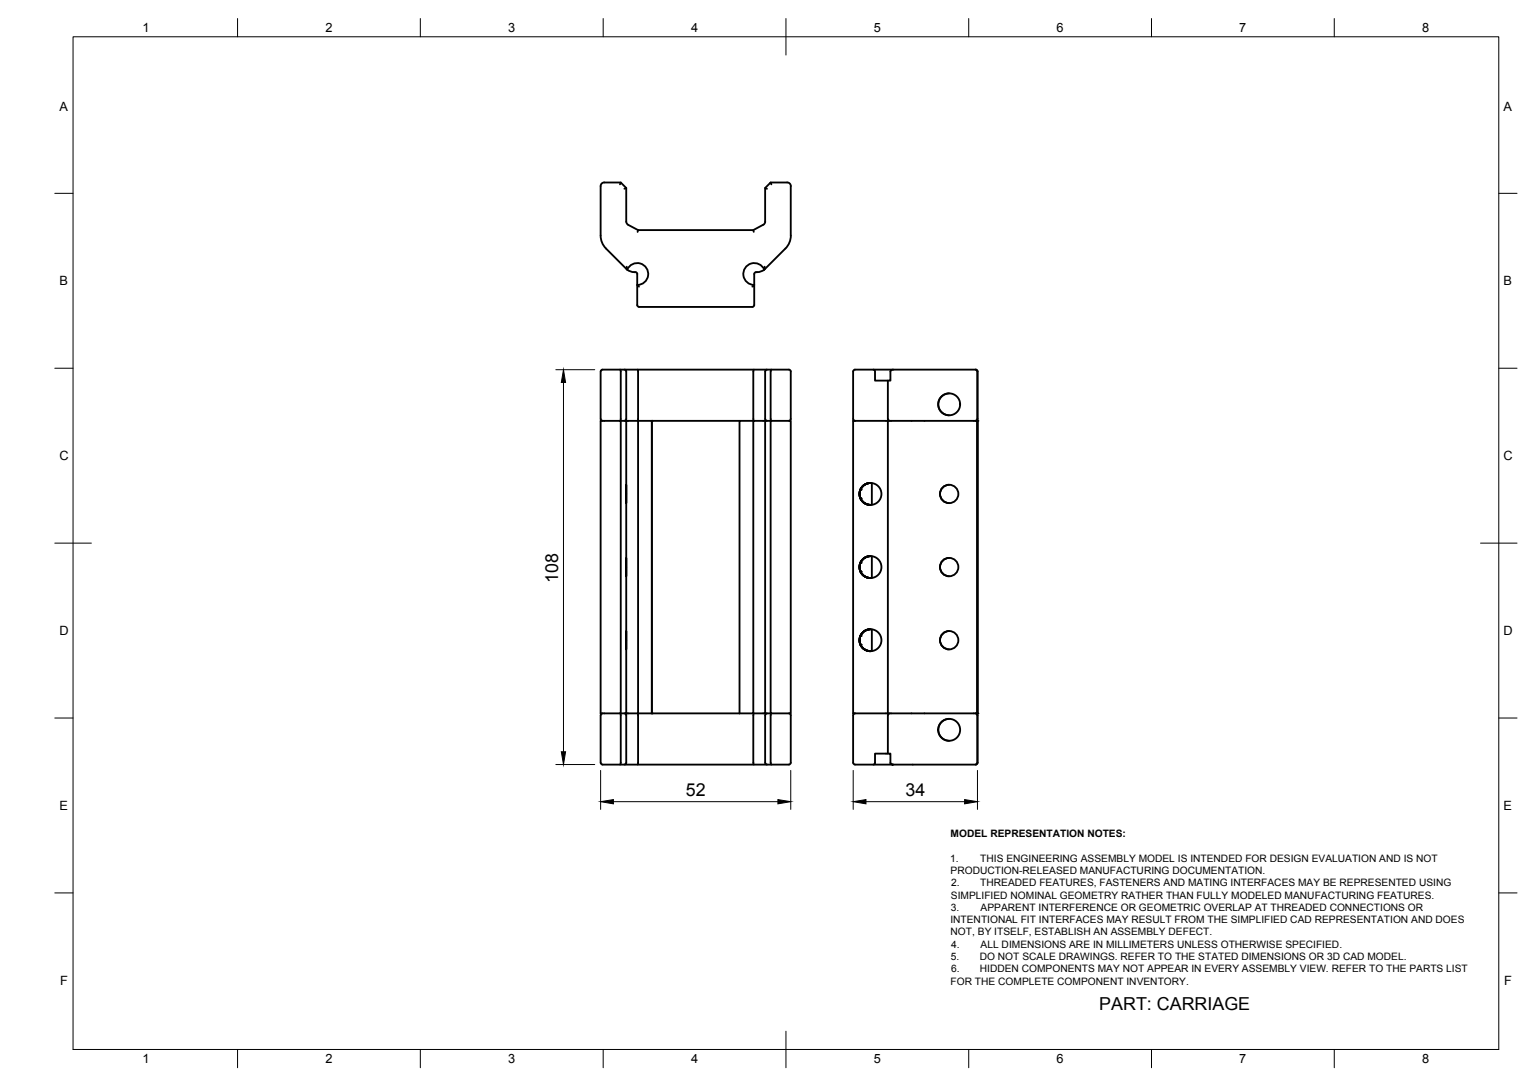
ISO-10303-21;
HEADER;
/* Generated by software containing ST-Developer
 * from STEP Tools, Inc. (www.steptools.com) 
 */

FILE_DESCRIPTION(
/* description */ (''),
/* implementation_level */ '2;1');

FILE_NAME(
/* name */ 'Carriage.step',
/* time_stamp */ '2026-10-05T11:01:41-07:00',
/* author */ (''),
/* organization */ (''),
/* preprocessor_version */ 'ST-DEVELOPER v20.2',
/* originating_system */ 'Autodesk Translation Framework v15.15.0.0',
/* authorisation */ '');

FILE_SCHEMA (('AUTOMOTIVE_DESIGN { 1 0 10303 214 3 1 1 }'));
ENDSEC;

DATA;
#10=MECHANICAL_DESIGN_GEOMETRIC_PRESENTATION_REPRESENTATION('',(#2142),#215609);
#119=ELLIPSE('',#29169,4.24264068711927,3.);
#120=ELLIPSE('',#29170,4.24264068711929,3.);
#121=ELLIPSE('',#29171,4.24264068711929,3.);
#122=ELLIPSE('',#29172,4.24279214221557,3.);
#123=ELLIPSE('',#29173,4.24279214221557,3.);
#124=ELLIPSE('',#29174,4.24248924824133,3.);
#125=ELLIPSE('',#29179,4.24248924824133,3.);
#126=ELLIPSE('',#29180,4.24279214221557,3.);
#127=ELLIPSE('',#29181,4.24264068711929,3.);
#128=ELLIPSE('',#29182,4.24264068711927,3.);
#129=ELLIPSE('',#29189,4.24264068711927,3.);
#130=ELLIPSE('',#29190,4.24264068711929,3.);
#131=ELLIPSE('',#29191,4.24264068711929,3.);
#132=ELLIPSE('',#29192,4.24279214221557,3.);
#133=ELLIPSE('',#29193,4.24279214221557,3.);
#134=ELLIPSE('',#29194,4.24248924824133,3.);
#135=ELLIPSE('',#29199,4.24248924824133,3.);
#136=ELLIPSE('',#29200,4.24279214221557,3.);
#137=ELLIPSE('',#29201,4.24264068711929,3.);
#138=ELLIPSE('',#29202,4.24264068711927,3.);
#139=ELLIPSE('',#29209,4.24264068711928,3.00000000000001);
#140=ELLIPSE('',#29210,4.24264068711931,3.00000000000001);
#141=ELLIPSE('',#29211,4.24264068711931,3.00000000000001);
#142=ELLIPSE('',#29212,4.24279214221559,3.00000000000001);
#143=ELLIPSE('',#29213,4.24279214221559,3.00000000000001);
#144=ELLIPSE('',#29214,4.24248924824134,3.00000000000001);
#145=ELLIPSE('',#29219,4.24248924824134,3.00000000000001);
#146=ELLIPSE('',#29220,4.24279214221559,3.00000000000001);
#147=ELLIPSE('',#29221,4.24264068711931,3.00000000000001);
#148=ELLIPSE('',#29222,4.24264068711928,3.00000000000001);
#204=FACE_BOUND('',#5046,.T.);
#205=FACE_BOUND('',#5047,.T.);
#206=FACE_BOUND('',#5048,.T.);
#207=FACE_BOUND('',#5055,.T.);
#208=FACE_BOUND('',#5056,.T.);
#209=FACE_BOUND('',#5057,.T.);
#210=FACE_BOUND('',#5062,.T.);
#211=FACE_BOUND('',#5063,.T.);
#212=FACE_BOUND('',#5064,.T.);
#213=FACE_BOUND('',#5089,.T.);
#214=FACE_BOUND('',#5090,.T.);
#215=FACE_BOUND('',#5091,.T.);
#1155=B_SPLINE_CURVE_WITH_KNOTS('',3,(#125658,#125659,#125660,#125661),
 .UNSPECIFIED.,.F.,.F.,(4,4),(0.425543658173478,0.45601992980538),
 .UNSPECIFIED.);
#1156=B_SPLINE_CURVE_WITH_KNOTS('',3,(#125665,#125666,#125667,#125668,#125669,
#125670,#125671,#125672,#125673,#125674),.UNSPECIFIED.,.F.,.F.,(4,2,2,2,
4),(-0.396099187348511,-0.387517388693499,-0.378935590038487,-0.34840050848607,
-0.288839883428953),.UNSPECIFIED.);
#1157=B_SPLINE_CURVE_WITH_KNOTS('',3,(#125678,#125679,#125680,#125681,#125682,
#125683,#125684,#125685,#125686,#125687,#125688,#125689,#125690,#125691,
#125692,#125693,#125694,#125695,#125696,#125697,#125698,#125699,#125700,
#125701,#125702,#125703),.UNSPECIFIED.,.F.,.F.,(4,2,2,2,2,2,2,2,2,2,2,2,
4),(0.255174199615659,0.258977839880058,0.262781480144458,0.270388760673256,
0.281246247196537,0.307084793231223,0.382761299423499,0.458437805615774,
0.484276351650461,0.495133838173742,0.50274111870254,0.506544758966939,
0.510348399231339),.UNSPECIFIED.);
#1158=B_SPLINE_CURVE_WITH_KNOTS('',3,(#125707,#125708,#125709,#125710,#125711,
#125712,#125713,#125714,#125715,#125716),.UNSPECIFIED.,.F.,.F.,(4,2,2,2,
4),(-0.107259303919562,-0.047698678862445,-0.0171635973100282,-0.00858179865501664,
-5.10702591327572E-15),.UNSPECIFIED.);
#1159=B_SPLINE_CURVE_WITH_KNOTS('',3,(#125720,#125721,#125722,#125723,#125724,
#125725),.UNSPECIFIED.,.F.,.F.,(4,2,4),(-0.229255666072561,-0.191461818559235,
-0.153667971045909),.UNSPECIFIED.);
#1160=B_SPLINE_CURVE_WITH_KNOTS('',3,(#125729,#125730,#125731,#125732,#125733,
#125734),.UNSPECIFIED.,.F.,.F.,(4,2,4),(-0.629374586597435,-0.551502061005561,
-0.473629535413688),.UNSPECIFIED.);
#1161=B_SPLINE_CURVE_WITH_KNOTS('',3,(#125738,#125739,#125740,#125741,#125742,
#125743),.UNSPECIFIED.,.F.,.F.,(4,2,4),(-2.19173462068589,-2.01009835047604,
-1.80563850045614),.UNSPECIFIED.);
#1162=B_SPLINE_CURVE_WITH_KNOTS('',3,(#125747,#125748,#125749,#125750,#125751,
#125752,#125753,#125754,#125755,#125756,#125757,#125758,#125759,#125760,
#125761,#125762),.UNSPECIFIED.,.F.,.F.,(4,2,2,2,2,2,2,4),(-0.591143586973193,
-0.574347005517868,-0.557550424062543,-0.523957261151894,-0.475997826184756,
-0.428038391217618,-0.391437431812971,-0.357248738805367),.UNSPECIFIED.);
#1163=B_SPLINE_CURVE_WITH_KNOTS('',3,(#125766,#125767,#125768,#125769,#125770,
#125771,#125772,#125773,#125774,#125775,#125776,#125777,#125778,#125779,
#125780,#125781,#125782,#125783,#125784,#125785,#125786,#125787,#125788,
#125789,#125790,#125791),.UNSPECIFIED.,.F.,.F.,(4,2,2,2,2,2,2,2,2,2,2,2,
4),(0.,0.00380879604231436,0.00761759208462871,0.0152351841692574,0.0261059417541897,
0.0519747072078825,0.127764798734132,0.203554890260381,0.229423655714074,
0.240294413299006,0.247912005383635,0.251720801425949,0.255529597468264),
 .UNSPECIFIED.);
#1164=B_SPLINE_CURVE_WITH_KNOTS('',3,(#125795,#125796,#125797,#125798,#125799,
#125800,#125801,#125802,#125803,#125804,#125805,#125806,#125807,#125808,
#125809,#125810),.UNSPECIFIED.,.F.,.F.,(4,2,2,2,2,2,2,4),(-0.233894848167829,
-0.199706155160222,-0.163105195755574,-0.115145760788437,-0.0671863258212992,
-0.0335931629106496,-0.0167965814553248,0.),.UNSPECIFIED.);
#1165=B_SPLINE_CURVE_WITH_KNOTS('',3,(#125818,#125819,#125820,#125821,#125822,
#125823,#125824,#125825,#125826,#125827,#125828,#125829,#125830,#125831,
#125832,#125833),.UNSPECIFIED.,.F.,.F.,(4,2,2,2,2,2,2,4),(-0.295589574301039,
-0.278794522803568,-0.261996615556423,-0.228400801062134,-0.180435395401912,
-0.13246998974169,-0.0958671986171408,-0.0616743717891369),
 .UNSPECIFIED.);
#1166=B_SPLINE_CURVE_WITH_KNOTS('',3,(#125837,#125838,#125839,#125840,#125841,
#125842,#125843,#125844,#125845,#125846,#125847,#125848,#125849,#125850,
#125851,#125852,#125853,#125854,#125855,#125856,#125857,#125858,#125859,
#125860,#125861,#125862),.UNSPECIFIED.,.F.,.F.,(4,2,2,2,2,2,2,2,2,2,2,2,
4),(0.255403168241683,0.259209043849209,0.263015990348529,0.270629883347168,
0.281495880894667,0.307353808398232,0.383103146024835,0.458852483651438,
0.484710411155003,0.495576408702502,0.503190301701141,0.506997248200461,
0.510803123807987),.UNSPECIFIED.);
#1167=B_SPLINE_CURVE_WITH_KNOTS('',3,(#125866,#125867,#125868,#125869,#125870,
#125871,#125872,#125873,#125874,#125875,#125876,#125877,#125878,#125879,
#125880,#125881),.UNSPECIFIED.,.F.,.F.,(4,2,2,2,2,2,2,4),(-0.525961887431026,
-0.491769060603023,-0.455166269478473,-0.407200863818251,-0.35923545815803,
-0.32563964366374,-0.308841736416595,-0.292046684919125),.UNSPECIFIED.);
#1168=B_SPLINE_CURVE_WITH_KNOTS('',3,(#125885,#125886,#125887,#125888,#125889,
#125890,#125891,#125892),.UNSPECIFIED.,.F.,.F.,(4,2,2,4),(-1.80557842881869,
-1.80556058066602,-1.60110476302328,-1.41948692443241),.UNSPECIFIED.);
#1169=B_SPLINE_CURVE_WITH_KNOTS('',3,(#125896,#125897,#125898,#125899,#125900,
#125901),.UNSPECIFIED.,.F.,.F.,(4,2,4),(-0.15576381568435,-0.0783128305768447,
-7.13925426615558E-6),.UNSPECIFIED.);
#1170=B_SPLINE_CURVE_WITH_KNOTS('',3,(#125905,#125906,#125907,#125908,#125909,
#125910,#125911,#125912,#125913,#125914),.UNSPECIFIED.,.F.,.F.,(4,2,2,2,
4),(-0.151179644005164,-0.151176055112586,-0.113501375709474,-0.0758266963063619,
-0.0755936744236418),.UNSPECIFIED.);
#1171=B_SPLINE_CURVE_WITH_KNOTS('',3,(#125918,#125919,#125920,#125921,#125922,
#125923,#125924,#125925,#125926,#125927,#125928,#125929,#125930,#125931),
 .UNSPECIFIED.,.F.,.F.,(4,2,2,2,2,2,4),(-0.199196015359092,-0.199194230558666,
-0.188883836185403,-0.17857344181214,-0.157952653065614,-0.123832754584569,
-0.0897155491016723),.UNSPECIFIED.);
#1172=B_SPLINE_CURVE_WITH_KNOTS('',3,(#125935,#125936,#125937,#125938,#125939,
#125940,#125941,#125942,#125943,#125944,#125945,#125946,#125947,#125948,
#125949,#125950,#125951,#125952,#125953,#125954,#125955,#125956,#125957,
#125958,#125959,#125960,#125961,#125962,#125963,#125964,#125965),
 .UNSPECIFIED.,.F.,.F.,(4,3,2,2,2,2,2,2,2,2,2,2,2,2,4),(0.509893253687354,
0.509894324579146,0.513694670705264,0.517495016831383,0.525095709083619,
0.535944713171104,0.561763938973776,0.637367905723932,0.712971872474088,
0.73879109827676,0.749640102364244,0.757240794616481,0.7610411407426,0.764841486868718,
0.764842557760511),.UNSPECIFIED.);
#1173=B_SPLINE_CURVE_WITH_KNOTS('',3,(#125969,#125970,#125971,#125972,#125973,
#125974,#125975,#125976,#125977,#125978,#125979,#125980,#125981,#125982),
 .UNSPECIFIED.,.F.,.F.,(4,2,2,2,2,2,4),(-0.306485394370277,-0.272368188887381,
-0.238248290406335,-0.217627501659809,-0.207317107286546,-0.197006712913283,
-0.197004928112857),.UNSPECIFIED.);
#1174=B_SPLINE_CURVE_WITH_KNOTS('',3,(#125986,#125987,#125988,#125989,#125990,
#125991),.UNSPECIFIED.,.F.,.F.,(4,2,4),(-0.489035198690406,-0.458517781350602,
-0.458514192458025),.UNSPECIFIED.);
#1175=B_SPLINE_CURVE_WITH_KNOTS('',3,(#125997,#125998,#125999,#126000,#126001,
#126002,#126003,#126004),.UNSPECIFIED.,.F.,.F.,(4,2,2,4),(-0.534100162039546,
-0.533867140156826,-0.496192460753714,-0.489035198690406),.UNSPECIFIED.);
#1176=B_SPLINE_CURVE_WITH_KNOTS('',3,(#126008,#126009,#126010,#126011,#126012,
#126013),.UNSPECIFIED.,.F.,.F.,(4,2,4),(-1.25873888352118,-1.1804331921986,
-1.10298220709109),.UNSPECIFIED.);
#1177=B_SPLINE_CURVE_WITH_KNOTS('',3,(#126017,#126018,#126019,#126020,#126021,
#126022,#126023,#126024,#126025),.UNSPECIFIED.,.F.,.F.,(4,2,3,4),(-0.386073656233604,
-0.204455817642737,0.,1.78481526716903E-5),.UNSPECIFIED.);
#1178=B_SPLINE_CURVE_WITH_KNOTS('',3,(#126030,#126031,#126032,#126033,#126034,
#126035),.UNSPECIFIED.,.F.,.F.,(4,2,4),(-3.61127700091229,-3.40681715089239,
-3.22518088068254),.UNSPECIFIED.);
#1179=B_SPLINE_CURVE_WITH_KNOTS('',3,(#126039,#126040,#126041,#126042,#126043,
#126044),.UNSPECIFIED.,.F.,.F.,(4,2,4),(-0.785102654344136,-0.707230128752262,
-0.629357603160389),.UNSPECIFIED.);
#1180=B_SPLINE_CURVE_WITH_KNOTS('',3,(#126047,#126048,#126049,#126050,#126051,
#126052),.UNSPECIFIED.,.F.,.F.,(4,2,4),(0.380432234778735,0.418226082292058,
0.425543658173478),.UNSPECIFIED.);
#1181=B_SPLINE_CURVE_WITH_KNOTS('',3,(#126064,#126065,#126066,#126067),
 .UNSPECIFIED.,.F.,.F.,(4,4),(0.425543658173478,0.45601992980538),
 .UNSPECIFIED.);
#1182=B_SPLINE_CURVE_WITH_KNOTS('',3,(#126071,#126072,#126073,#126074,#126075,
#126076,#126077,#126078,#126079,#126080),.UNSPECIFIED.,.F.,.F.,(4,2,2,2,
4),(-0.396099187348511,-0.387517388693499,-0.378935590038488,-0.348400508486071,
-0.288839883428954),.UNSPECIFIED.);
#1183=B_SPLINE_CURVE_WITH_KNOTS('',3,(#126084,#126085,#126086,#126087,#126088,
#126089,#126090,#126091,#126092,#126093,#126094,#126095,#126096,#126097,
#126098,#126099,#126100,#126101,#126102,#126103,#126104,#126105,#126106,
#126107,#126108,#126109),.UNSPECIFIED.,.F.,.F.,(4,2,2,2,2,2,2,2,2,2,2,2,
4),(0.255174199615659,0.258977839880058,0.262781480144457,0.270388760673256,
0.281246247196536,0.307084793231223,0.382761299423499,0.458437805615774,
0.48427635165046,0.495133838173741,0.50274111870254,0.506544758966939,0.510348399231338),
 .UNSPECIFIED.);
#1184=B_SPLINE_CURVE_WITH_KNOTS('',3,(#126113,#126114,#126115,#126116,#126117,
#126118,#126119,#126120,#126121,#126122),.UNSPECIFIED.,.F.,.F.,(4,2,2,2,
4),(-0.107259303919562,-0.047698678862445,-0.0171635973100282,-0.00858179865501664,
-5.10702591327572E-15),.UNSPECIFIED.);
#1185=B_SPLINE_CURVE_WITH_KNOTS('',3,(#126126,#126127,#126128,#126129,#126130,
#126131),.UNSPECIFIED.,.F.,.F.,(4,2,4),(-0.229255666072561,-0.191461818559235,
-0.153667971045909),.UNSPECIFIED.);
#1186=B_SPLINE_CURVE_WITH_KNOTS('',3,(#126135,#126136,#126137,#126138,#126139,
#126140),.UNSPECIFIED.,.F.,.F.,(4,2,4),(-0.629374586597435,-0.551502061005562,
-0.47362953541369),.UNSPECIFIED.);
#1187=B_SPLINE_CURVE_WITH_KNOTS('',3,(#126144,#126145,#126146,#126147,#126148,
#126149),.UNSPECIFIED.,.F.,.F.,(4,2,4),(-2.19173462068589,-2.01009835047603,
-1.80563850045614),.UNSPECIFIED.);
#1188=B_SPLINE_CURVE_WITH_KNOTS('',3,(#126153,#126154,#126155,#126156,#126157,
#126158,#126159,#126160,#126161,#126162,#126163,#126164,#126165,#126166,
#126167,#126168),.UNSPECIFIED.,.F.,.F.,(4,2,2,2,2,2,2,4),(-0.591143586973193,
-0.574347005517868,-0.557550424062543,-0.523957261151894,-0.475997826184756,
-0.428038391217618,-0.391437431812971,-0.357248738805362),.UNSPECIFIED.);
#1189=B_SPLINE_CURVE_WITH_KNOTS('',3,(#126172,#126173,#126174,#126175,#126176,
#126177,#126178,#126179,#126180,#126181,#126182,#126183,#126184,#126185,
#126186,#126187,#126188,#126189,#126190,#126191,#126192,#126193,#126194,
#126195,#126196,#126197),.UNSPECIFIED.,.F.,.F.,(4,2,2,2,2,2,2,2,2,2,2,2,
4),(0.,0.00380879604231436,0.00761759208462871,0.0152351841692574,0.0261059417541897,
0.0519747072078817,0.127764798734132,0.203554890260381,0.229423655714074,
0.240294413299006,0.247912005383635,0.251720801425949,0.255529597468264),
 .UNSPECIFIED.);
#1190=B_SPLINE_CURVE_WITH_KNOTS('',3,(#126201,#126202,#126203,#126204,#126205,
#126206,#126207,#126208,#126209,#126210,#126211,#126212,#126213,#126214,
#126215,#126216),.UNSPECIFIED.,.F.,.F.,(4,2,2,2,2,2,2,4),(-0.233894848167831,
-0.199706155160222,-0.163105195755574,-0.115145760788437,-0.0671863258212992,
-0.0335931629106496,-0.0167965814553248,0.),.UNSPECIFIED.);
#1191=B_SPLINE_CURVE_WITH_KNOTS('',3,(#126224,#126225,#126226,#126227,#126228,
#126229,#126230,#126231,#126232,#126233,#126234,#126235,#126236,#126237,
#126238,#126239),.UNSPECIFIED.,.F.,.F.,(4,2,2,2,2,2,2,4),(-0.295589574301039,
-0.278794522803568,-0.261996615556423,-0.228400801062134,-0.180435395401912,
-0.13246998974169,-0.0958671986171408,-0.0616743717891374),
 .UNSPECIFIED.);
#1192=B_SPLINE_CURVE_WITH_KNOTS('',3,(#126243,#126244,#126245,#126246,#126247,
#126248,#126249,#126250,#126251,#126252,#126253,#126254,#126255,#126256,
#126257,#126258,#126259,#126260,#126261,#126262,#126263,#126264,#126265,
#126266,#126267,#126268),.UNSPECIFIED.,.F.,.F.,(4,2,2,2,2,2,2,2,2,2,2,2,
4),(0.255403168241683,0.259209043849209,0.263015990348529,0.270629883347168,
0.281495880894667,0.307353808398233,0.383103146024836,0.458852483651437,
0.484710411155004,0.495576408702501,0.503190301701141,0.50699724820046,
0.510803123807986),.UNSPECIFIED.);
#1193=B_SPLINE_CURVE_WITH_KNOTS('',3,(#126272,#126273,#126274,#126275,#126276,
#126277,#126278,#126279,#126280,#126281,#126282,#126283,#126284,#126285,
#126286,#126287),.UNSPECIFIED.,.F.,.F.,(4,2,2,2,2,2,2,4),(-0.525961887431026,
-0.491769060603023,-0.455166269478473,-0.407200863818251,-0.35923545815803,
-0.32563964366374,-0.308841736416595,-0.292046684919125),.UNSPECIFIED.);
#1194=B_SPLINE_CURVE_WITH_KNOTS('',3,(#126291,#126292,#126293,#126294,#126295,
#126296,#126297,#126298),.UNSPECIFIED.,.F.,.F.,(4,2,2,4),(-1.80557842881869,
-1.80556058066602,-1.60110476302328,-1.41948692443241),.UNSPECIFIED.);
#1195=B_SPLINE_CURVE_WITH_KNOTS('',3,(#126302,#126303,#126304,#126305,#126306,
#126307),.UNSPECIFIED.,.F.,.F.,(4,2,4),(-0.15576381568435,-0.0783128305768447,
-7.13925426615561E-6),.UNSPECIFIED.);
#1196=B_SPLINE_CURVE_WITH_KNOTS('',3,(#126311,#126312,#126313,#126314,#126315,
#126316,#126317,#126318,#126319,#126320),.UNSPECIFIED.,.F.,.F.,(4,2,2,2,
4),(-0.151179644005162,-0.151176055112586,-0.113501375709474,-0.0758266963063619,
-0.0755936744236418),.UNSPECIFIED.);
#1197=B_SPLINE_CURVE_WITH_KNOTS('',3,(#126324,#126325,#126326,#126327,#126328,
#126329,#126330,#126331,#126332,#126333,#126334,#126335,#126336,#126337),
 .UNSPECIFIED.,.F.,.F.,(4,2,2,2,2,2,4),(-0.199196015359092,-0.199194230558666,
-0.188883836185403,-0.17857344181214,-0.157952653065614,-0.123832754584569,
-0.0897155491016734),.UNSPECIFIED.);
#1198=B_SPLINE_CURVE_WITH_KNOTS('',3,(#126341,#126342,#126343,#126344,#126345,
#126346,#126347,#126348,#126349,#126350,#126351,#126352,#126353,#126354,
#126355,#126356,#126357,#126358,#126359,#126360,#126361,#126362,#126363,
#126364,#126365,#126366,#126367,#126368,#126369,#126370,#126371),
 .UNSPECIFIED.,.F.,.F.,(4,3,2,2,2,2,2,2,2,2,2,2,2,2,4),(0.509893253687354,
0.509894324579146,0.513694670705264,0.517495016831383,0.525095709083619,
0.535944713171104,0.561763938973776,0.637367905723932,0.712971872474088,
0.73879109827676,0.749640102364244,0.757240794616481,0.7610411407426,0.764841486868718,
0.764842557760511),.UNSPECIFIED.);
#1199=B_SPLINE_CURVE_WITH_KNOTS('',3,(#126375,#126376,#126377,#126378,#126379,
#126380,#126381,#126382,#126383,#126384,#126385,#126386,#126387,#126388),
 .UNSPECIFIED.,.F.,.F.,(4,2,2,2,2,2,4),(-0.306485394370277,-0.272368188887381,
-0.238248290406335,-0.217627501659809,-0.207317107286546,-0.197006712913283,
-0.197004928112857),.UNSPECIFIED.);
#1200=B_SPLINE_CURVE_WITH_KNOTS('',3,(#126392,#126393,#126394,#126395,#126396,
#126397),.UNSPECIFIED.,.F.,.F.,(4,2,4),(-0.489035198690406,-0.458517781350602,
-0.458514192458025),.UNSPECIFIED.);
#1201=B_SPLINE_CURVE_WITH_KNOTS('',3,(#126403,#126404,#126405,#126406,#126407,
#126408,#126409,#126410),.UNSPECIFIED.,.F.,.F.,(4,2,2,4),(-0.534100162039546,
-0.533867140156826,-0.496192460753714,-0.489035198690406),.UNSPECIFIED.);
#1202=B_SPLINE_CURVE_WITH_KNOTS('',3,(#126414,#126415,#126416,#126417,#126418,
#126419),.UNSPECIFIED.,.F.,.F.,(4,2,4),(-1.25873888352118,-1.1804331921986,
-1.10298220709109),.UNSPECIFIED.);
#1203=B_SPLINE_CURVE_WITH_KNOTS('',3,(#126423,#126424,#126425,#126426,#126427,
#126428,#126429,#126430,#126431),.UNSPECIFIED.,.F.,.F.,(4,2,3,4),(-0.386073656233604,
-0.204455817642737,0.,1.78481526716903E-5),.UNSPECIFIED.);
#1204=B_SPLINE_CURVE_WITH_KNOTS('',3,(#126436,#126437,#126438,#126439,#126440,
#126441),.UNSPECIFIED.,.F.,.F.,(4,2,4),(-3.61127700091229,-3.40681715089239,
-3.22518088068254),.UNSPECIFIED.);
#1205=B_SPLINE_CURVE_WITH_KNOTS('',3,(#126445,#126446,#126447,#126448,#126449,
#126450),.UNSPECIFIED.,.F.,.F.,(4,2,4),(-0.785102654344136,-0.707230128752262,
-0.629357603160389),.UNSPECIFIED.);
#1206=B_SPLINE_CURVE_WITH_KNOTS('',3,(#126453,#126454,#126455,#126456,#126457,
#126458),.UNSPECIFIED.,.F.,.F.,(4,2,4),(0.380432234778735,0.418226082292058,
0.425543658173478),.UNSPECIFIED.);
#1207=B_SPLINE_CURVE_WITH_KNOTS('',3,(#126470,#126471,#126472,#126473),
 .UNSPECIFIED.,.F.,.F.,(4,4),(0.425543658173479,0.45601992980538),
 .UNSPECIFIED.);
#1208=B_SPLINE_CURVE_WITH_KNOTS('',3,(#126477,#126478,#126479,#126480,#126481,
#126482,#126483,#126484,#126485,#126486,#126487,#126488),.UNSPECIFIED.,
 .F.,.F.,(4,2,2,2,2,4),(-0.398283608397278,-0.387975515458133,-0.377667422518988,
-0.357051236640699,-0.322947181787487,-0.288843126934276),.UNSPECIFIED.);
#1209=B_SPLINE_CURVE_WITH_KNOTS('',3,(#126492,#126493,#126494,#126495,#126496,
#126497,#126498,#126499,#126500,#126501,#126502,#126503,#126504,#126505,
#126506,#126507,#126508,#126509,#126510,#126511,#126512,#126513,#126514,
#126515,#126516,#126517),.UNSPECIFIED.,.F.,.F.,(4,2,2,2,2,2,2,2,2,2,2,2,
4),(0.255174199615664,0.258977839880064,0.262781480144463,0.270388760673262,
0.281246247196542,0.307084793231227,0.382761299423505,0.458437805615783,
0.484276351650471,0.495133838173751,0.50274111870255,0.50654475896695,0.510348399231349),
 .UNSPECIFIED.);
#1210=B_SPLINE_CURVE_WITH_KNOTS('',3,(#126521,#126522,#126523,#126524,#126525,
#126526,#126527,#126528,#126529,#126530,#126531,#126532),.UNSPECIFIED.,
 .F.,.F.,(4,2,2,2,2,4),(-0.109440481463008,-0.075336426609796,-0.0412323717565842,
-0.0206161858782945,-0.0103080929391497,-4.88498130835069E-15),
 .UNSPECIFIED.);
#1211=B_SPLINE_CURVE_WITH_KNOTS('',3,(#126536,#126537,#126538,#126539,#126540,
#126541),.UNSPECIFIED.,.F.,.F.,(4,2,4),(-0.229255666072554,-0.191461818559231,
-0.153667971045908),.UNSPECIFIED.);
#1212=B_SPLINE_CURVE_WITH_KNOTS('',3,(#126545,#126546,#126547,#126548,#126549,
#126550),.UNSPECIFIED.,.F.,.F.,(4,2,4),(-0.629374586597435,-0.551502061005562,
-0.473629535413688),.UNSPECIFIED.);
#1213=B_SPLINE_CURVE_WITH_KNOTS('',3,(#126554,#126555,#126556,#126557,#126558,
#126559),.UNSPECIFIED.,.F.,.F.,(4,2,4),(-2.19173462068589,-2.01009835047604,
-1.80563850045615),.UNSPECIFIED.);
#1214=B_SPLINE_CURVE_WITH_KNOTS('',3,(#126563,#126564,#126565,#126566,#126567,
#126568,#126569,#126570,#126571,#126572,#126573,#126574,#126575,#126576,
#126577,#126578),.UNSPECIFIED.,.F.,.F.,(4,2,2,2,2,2,2,4),(-0.591143586973191,
-0.574347005517867,-0.557550424062542,-0.523957261151894,-0.475997826184755,
-0.428038391217617,-0.391437431812969,-0.357248738805361),.UNSPECIFIED.);
#1215=B_SPLINE_CURVE_WITH_KNOTS('',3,(#126582,#126583,#126584,#126585,#126586,
#126587,#126588,#126589,#126590,#126591,#126592,#126593,#126594,#126595,
#126596,#126597,#126598,#126599,#126600,#126601,#126602,#126603,#126604,
#126605,#126606,#126607),.UNSPECIFIED.,.F.,.F.,(4,2,2,2,2,2,2,2,2,2,2,2,
4),(0.,0.00380879604231454,0.00761759208462907,0.0152351841692581,0.0261059417541897,
0.0519747072078822,0.127764798734136,0.203554890260386,0.22942365571408,
0.240294413299011,0.24791200538364,0.251720801425955,0.255529597468269),
 .UNSPECIFIED.);
#1216=B_SPLINE_CURVE_WITH_KNOTS('',3,(#126611,#126612,#126613,#126614,#126615,
#126616,#126617,#126618,#126619,#126620,#126621,#126622,#126623,#126624,
#126625,#126626),.UNSPECIFIED.,.F.,.F.,(4,2,2,2,2,2,2,4),(-0.233894848167828,
-0.199706155160221,-0.163105195755574,-0.115145760788435,-0.0671863258212968,
-0.0335931629106484,-0.0167965814553242,0.),.UNSPECIFIED.);
#1217=B_SPLINE_CURVE_WITH_KNOTS('',3,(#126634,#126635,#126636,#126637,#126638,
#126639,#126640,#126641,#126642,#126643,#126644,#126645,#126646,#126647,
#126648,#126649),.UNSPECIFIED.,.F.,.F.,(4,2,2,2,2,2,2,4),(-0.295589574301038,
-0.278794522803567,-0.261996615556422,-0.228400801062133,-0.180435395401912,
-0.132469989741691,-0.095867198617141,-0.0616743717891376),
 .UNSPECIFIED.);
#1218=B_SPLINE_CURVE_WITH_KNOTS('',3,(#126653,#126654,#126655,#126656,#126657,
#126658,#126659,#126660,#126661,#126662,#126663,#126664,#126665,#126666,
#126667,#126668,#126669,#126670,#126671,#126672,#126673,#126674,#126675,
#126676,#126677,#126678),.UNSPECIFIED.,.F.,.F.,(4,2,2,2,2,2,2,2,2,2,2,2,
4),(0.255403168241688,0.259209043849214,0.263015990348534,0.270629883347173,
0.281495880894669,0.307353808398237,0.38310314602484,0.458852483651447,
0.484710411155011,0.495576408702511,0.50319030170115,0.506997248200469,
0.510803123807995),.UNSPECIFIED.);
#1219=B_SPLINE_CURVE_WITH_KNOTS('',3,(#126682,#126683,#126684,#126685,#126686,
#126687,#126688,#126689,#126690,#126691,#126692,#126693,#126694,#126695,
#126696,#126697),.UNSPECIFIED.,.F.,.F.,(4,2,2,2,2,2,2,4),(-0.525961887431025,
-0.491769060603021,-0.455166269478471,-0.40720086381825,-0.359235458158029,
-0.32563964366374,-0.308841736416595,-0.292046684919124),.UNSPECIFIED.);
#1220=B_SPLINE_CURVE_WITH_KNOTS('',3,(#126701,#126702,#126703,#126704,#126705,
#126706,#126707,#126708),.UNSPECIFIED.,.F.,.F.,(4,2,2,4),(-1.80557842881869,
-1.80556058066602,-1.60110476302328,-1.41948692443242),.UNSPECIFIED.);
#1221=B_SPLINE_CURVE_WITH_KNOTS('',3,(#126712,#126713,#126714,#126715,#126716,
#126717),.UNSPECIFIED.,.F.,.F.,(4,2,4),(-0.155763815684349,-0.0783128305768452,
-7.13925426615562E-6),.UNSPECIFIED.);
#1222=B_SPLINE_CURVE_WITH_KNOTS('',3,(#126721,#126722,#126723,#126724,#126725,
#126726,#126727,#126728,#126729,#126730),.UNSPECIFIED.,.F.,.F.,(4,2,2,2,
4),(-0.151179644004872,-0.151176055112587,-0.113501375709475,-0.0758266963063625,
-0.0755936744236423),.UNSPECIFIED.);
#1223=B_SPLINE_CURVE_WITH_KNOTS('',3,(#126734,#126735,#126736,#126737,#126738,
#126739,#126740,#126741,#126742,#126743,#126744,#126745,#126746,#126747),
 .UNSPECIFIED.,.F.,.F.,(4,2,2,2,2,2,4),(-0.199196015359092,-0.199194230558666,
-0.188883836185403,-0.178573441812139,-0.157952653065613,-0.123832754584568,
-0.0897155491016729),.UNSPECIFIED.);
#1224=B_SPLINE_CURVE_WITH_KNOTS('',3,(#126751,#126752,#126753,#126754,#126755,
#126756,#126757,#126758,#126759,#126760,#126761,#126762,#126763,#126764,
#126765,#126766,#126767,#126768,#126769,#126770,#126771,#126772,#126773,
#126774,#126775,#126776,#126777,#126778,#126779,#126780,#126781),
 .UNSPECIFIED.,.F.,.F.,(4,3,2,2,2,2,2,2,2,2,2,2,2,2,4),(0.509893253687361,
0.509894324579153,0.513694670705272,0.51749501683139,0.525095709083628,
0.535944713171112,0.561763938973786,0.637367905723943,0.7129718724741,0.738791098276774,
0.749640102364255,0.757240794616493,0.761041140742611,0.76484148686873,
0.764842557760522),.UNSPECIFIED.);
#1225=B_SPLINE_CURVE_WITH_KNOTS('',3,(#126785,#126786,#126787,#126788,#126789,
#126790,#126791,#126792,#126793,#126794,#126795,#126796,#126797,#126798),
 .UNSPECIFIED.,.F.,.F.,(4,2,2,2,2,2,4),(-0.306485394370274,-0.27236818888738,
-0.238248290406335,-0.217627501659809,-0.207317107286546,-0.197006712913282,
-0.197004928112857),.UNSPECIFIED.);
#1226=B_SPLINE_CURVE_WITH_KNOTS('',3,(#126802,#126803,#126804,#126805,#126806,
#126807),.UNSPECIFIED.,.F.,.F.,(4,2,4),(-0.489034960252788,-0.458517542912984,
-0.458513954020698),.UNSPECIFIED.);
#1227=B_SPLINE_CURVE_WITH_KNOTS('',3,(#126813,#126814,#126815,#126816,#126817,
#126818,#126819,#126820),.UNSPECIFIED.,.F.,.F.,(4,2,2,4),(-0.534099923601928,
-0.533866901719208,-0.496192222316096,-0.489034960252788),.UNSPECIFIED.);
#1228=B_SPLINE_CURVE_WITH_KNOTS('',3,(#126824,#126825,#126826,#126827,#126828,
#126829),.UNSPECIFIED.,.F.,.F.,(4,2,4),(-1.25874265108256,-1.18043695975999,
-1.10298597465248),.UNSPECIFIED.);
#1229=B_SPLINE_CURVE_WITH_KNOTS('',3,(#126833,#126834,#126835,#126836,#126837,
#126838,#126839,#126840,#126841),.UNSPECIFIED.,.F.,.F.,(4,2,3,4),(-0.386073656233605,
-0.204455817642737,0.,1.78481526712462E-5),.UNSPECIFIED.);
#1230=B_SPLINE_CURVE_WITH_KNOTS('',3,(#126846,#126847,#126848,#126849,#126850,
#126851),.UNSPECIFIED.,.F.,.F.,(4,2,4),(-3.6112770009123,-3.4068171508924,
-3.22518088068255),.UNSPECIFIED.);
#1231=B_SPLINE_CURVE_WITH_KNOTS('',3,(#126855,#126856,#126857,#126858,#126859,
#126860),.UNSPECIFIED.,.F.,.F.,(4,2,4),(-0.785102654344135,-0.707230128752262,
-0.62935760316039),.UNSPECIFIED.);
#1232=B_SPLINE_CURVE_WITH_KNOTS('',3,(#126863,#126864,#126865,#126866,#126867,
#126868),.UNSPECIFIED.,.F.,.F.,(4,2,4),(0.380432234778735,0.418226082292058,
0.425543658173479),.UNSPECIFIED.);
#2124=SHAPE_REPRESENTATION_RELATIONSHIP('SRR','None',#215647,#2133);
#2133=ADVANCED_BREP_SHAPE_REPRESENTATION('',(#2151),#215603);
#2142=STYLED_ITEM('',(#215698),#2151);
#2151=MANIFOLD_SOLID_BREP('Body1',#28085);
#2564=CYLINDRICAL_SURFACE('',#29152,3.);
#2565=CYLINDRICAL_SURFACE('',#29157,3.00000000000001);
#2566=CYLINDRICAL_SURFACE('',#29165,3.);
#2567=CYLINDRICAL_SURFACE('',#29185,3.);
#2568=CYLINDRICAL_SURFACE('',#29205,3.00000000000001);
#2569=CYLINDRICAL_SURFACE('',#29223,0.3);
#2570=CYLINDRICAL_SURFACE('',#29229,0.499999999999998);
#2571=CYLINDRICAL_SURFACE('',#29231,0.499999999999998);
#2572=CYLINDRICAL_SURFACE('',#29233,0.499999999999998);
#2573=CYLINDRICAL_SURFACE('',#29237,1.);
#2574=CYLINDRICAL_SURFACE('',#29239,1.);
#2575=CYLINDRICAL_SURFACE('',#29241,1.);
#2576=CYLINDRICAL_SURFACE('',#29245,2.);
#2577=CYLINDRICAL_SURFACE('',#29247,2.);
#2578=CYLINDRICAL_SURFACE('',#29249,2.);
#2579=CYLINDRICAL_SURFACE('',#29253,5.);
#2580=CYLINDRICAL_SURFACE('',#29255,5.);
#2581=CYLINDRICAL_SURFACE('',#29257,5.);
#2582=CYLINDRICAL_SURFACE('',#29261,0.800000000000001);
#2583=CYLINDRICAL_SURFACE('',#29263,0.800000000000001);
#2584=CYLINDRICAL_SURFACE('',#29265,0.800000000000001);
#2585=CYLINDRICAL_SURFACE('',#29269,0.3);
#2586=CYLINDRICAL_SURFACE('',#29275,0.499999999999998);
#2587=CYLINDRICAL_SURFACE('',#29277,0.499999999999998);
#2588=CYLINDRICAL_SURFACE('',#29278,0.499999999999998);
#2589=CYLINDRICAL_SURFACE('',#29282,1.);
#2590=CYLINDRICAL_SURFACE('',#29284,1.);
#2591=CYLINDRICAL_SURFACE('',#29285,1.);
#2592=CYLINDRICAL_SURFACE('',#29289,2.);
#2593=CYLINDRICAL_SURFACE('',#29291,2.);
#2594=CYLINDRICAL_SURFACE('',#29292,2.);
#2595=CYLINDRICAL_SURFACE('',#29296,5.);
#2596=CYLINDRICAL_SURFACE('',#29298,5.);
#2597=CYLINDRICAL_SURFACE('',#29299,5.);
#2598=CYLINDRICAL_SURFACE('',#29303,0.800000000000001);
#2599=CYLINDRICAL_SURFACE('',#29305,0.800000000000001);
#2600=CYLINDRICAL_SURFACE('',#29306,0.800000000000001);
#2601=CYLINDRICAL_SURFACE('',#29310,2.5);
#2602=CYLINDRICAL_SURFACE('',#29313,2.5);
#2603=CYLINDRICAL_SURFACE('',#29316,2.5);
#2604=CYLINDRICAL_SURFACE('',#29321,0.3);
#2605=CYLINDRICAL_SURFACE('',#29325,0.300000000000002);
#2606=CYLINDRICAL_SURFACE('',#29329,0.800000000000001);
#2607=CYLINDRICAL_SURFACE('',#29331,5.);
#2608=CYLINDRICAL_SURFACE('',#29333,2.);
#2609=CYLINDRICAL_SURFACE('',#29335,1.);
#2610=CYLINDRICAL_SURFACE('',#29337,0.499999999999998);
#2611=CYLINDRICAL_SURFACE('',#29340,0.300000000000002);
#2612=CYLINDRICAL_SURFACE('',#29344,0.500000000000001);
#2613=CYLINDRICAL_SURFACE('',#29348,0.508000000000002);
#2614=CYLINDRICAL_SURFACE('',#29352,3.);
#2615=CYLINDRICAL_SURFACE('',#29356,5.);
#2616=CYLINDRICAL_SURFACE('',#29360,1.);
#2617=CYLINDRICAL_SURFACE('',#29366,1.);
#2618=CYLINDRICAL_SURFACE('',#29373,0.3);
#2619=CYLINDRICAL_SURFACE('',#29377,0.300000000000002);
#2620=CYLINDRICAL_SURFACE('',#29381,0.800000000000001);
#2621=CYLINDRICAL_SURFACE('',#29384,5.);
#2622=CYLINDRICAL_SURFACE('',#29387,2.);
#2623=CYLINDRICAL_SURFACE('',#29390,1.);
#2624=CYLINDRICAL_SURFACE('',#29393,0.499999999999998);
#2625=CYLINDRICAL_SURFACE('',#29397,0.300000000000002);
#2626=CYLINDRICAL_SURFACE('',#29401,0.5);
#2627=CYLINDRICAL_SURFACE('',#29405,0.508000000000002);
#2628=CYLINDRICAL_SURFACE('',#29409,3.);
#2629=CYLINDRICAL_SURFACE('',#29413,5.);
#2630=CYLINDRICAL_SURFACE('',#29417,1.);
#2631=CYLINDRICAL_SURFACE('',#29423,1.);
#3599=FACE_OUTER_BOUND('',#4943,.T.);
#3600=FACE_OUTER_BOUND('',#4944,.T.);
#3601=FACE_OUTER_BOUND('',#4945,.T.);
#3602=FACE_OUTER_BOUND('',#4946,.T.);
#3603=FACE_OUTER_BOUND('',#4947,.T.);
#3604=FACE_OUTER_BOUND('',#4948,.T.);
#3605=FACE_OUTER_BOUND('',#4949,.T.);
#3606=FACE_OUTER_BOUND('',#4950,.T.);
#3607=FACE_OUTER_BOUND('',#4951,.T.);
#3608=FACE_OUTER_BOUND('',#4952,.T.);
#3609=FACE_OUTER_BOUND('',#4953,.T.);
#3610=FACE_OUTER_BOUND('',#4954,.T.);
#3611=FACE_OUTER_BOUND('',#4955,.T.);
#3612=FACE_OUTER_BOUND('',#4956,.T.);
#3613=FACE_OUTER_BOUND('',#4957,.T.);
#3614=FACE_OUTER_BOUND('',#4958,.T.);
#3615=FACE_OUTER_BOUND('',#4959,.T.);
#3616=FACE_OUTER_BOUND('',#4960,.T.);
#3617=FACE_OUTER_BOUND('',#4961,.T.);
#3618=FACE_OUTER_BOUND('',#4962,.T.);
#3619=FACE_OUTER_BOUND('',#4963,.T.);
#3620=FACE_OUTER_BOUND('',#4964,.T.);
#3621=FACE_OUTER_BOUND('',#4965,.T.);
#3622=FACE_OUTER_BOUND('',#4966,.T.);
#3623=FACE_OUTER_BOUND('',#4967,.T.);
#3624=FACE_OUTER_BOUND('',#4968,.T.);
#3625=FACE_OUTER_BOUND('',#4969,.T.);
#3626=FACE_OUTER_BOUND('',#4970,.T.);
#3627=FACE_OUTER_BOUND('',#4971,.T.);
#3628=FACE_OUTER_BOUND('',#4972,.T.);
#3629=FACE_OUTER_BOUND('',#4973,.T.);
#3630=FACE_OUTER_BOUND('',#4974,.T.);
#3631=FACE_OUTER_BOUND('',#4975,.T.);
#3632=FACE_OUTER_BOUND('',#4976,.T.);
#3633=FACE_OUTER_BOUND('',#4977,.T.);
#3634=FACE_OUTER_BOUND('',#4978,.T.);
#3635=FACE_OUTER_BOUND('',#4979,.T.);
#3636=FACE_OUTER_BOUND('',#4980,.T.);
#3637=FACE_OUTER_BOUND('',#4981,.T.);
#3638=FACE_OUTER_BOUND('',#4982,.T.);
#3639=FACE_OUTER_BOUND('',#4983,.T.);
#3640=FACE_OUTER_BOUND('',#4984,.T.);
#3641=FACE_OUTER_BOUND('',#4985,.T.);
#3642=FACE_OUTER_BOUND('',#4986,.T.);
#3643=FACE_OUTER_BOUND('',#4987,.T.);
#3644=FACE_OUTER_BOUND('',#4988,.T.);
#3645=FACE_OUTER_BOUND('',#4989,.T.);
#3646=FACE_OUTER_BOUND('',#4990,.T.);
#3647=FACE_OUTER_BOUND('',#4991,.T.);
#3648=FACE_OUTER_BOUND('',#4992,.T.);
#3649=FACE_OUTER_BOUND('',#4993,.T.);
#3650=FACE_OUTER_BOUND('',#4994,.T.);
#3651=FACE_OUTER_BOUND('',#4995,.T.);
#3652=FACE_OUTER_BOUND('',#4996,.T.);
#3653=FACE_OUTER_BOUND('',#4997,.T.);
#3654=FACE_OUTER_BOUND('',#4998,.T.);
#3655=FACE_OUTER_BOUND('',#4999,.T.);
#3656=FACE_OUTER_BOUND('',#5000,.T.);
#3657=FACE_OUTER_BOUND('',#5001,.T.);
#3658=FACE_OUTER_BOUND('',#5002,.T.);
#3659=FACE_OUTER_BOUND('',#5003,.T.);
#3660=FACE_OUTER_BOUND('',#5004,.T.);
#3661=FACE_OUTER_BOUND('',#5005,.T.);
#3662=FACE_OUTER_BOUND('',#5006,.T.);
#3663=FACE_OUTER_BOUND('',#5007,.T.);
#3664=FACE_OUTER_BOUND('',#5008,.T.);
#3665=FACE_OUTER_BOUND('',#5009,.T.);
#3666=FACE_OUTER_BOUND('',#5010,.T.);
#3667=FACE_OUTER_BOUND('',#5011,.T.);
#3668=FACE_OUTER_BOUND('',#5012,.T.);
#3669=FACE_OUTER_BOUND('',#5013,.T.);
#3670=FACE_OUTER_BOUND('',#5014,.T.);
#3671=FACE_OUTER_BOUND('',#5015,.T.);
#3672=FACE_OUTER_BOUND('',#5016,.T.);
#3673=FACE_OUTER_BOUND('',#5017,.T.);
#3674=FACE_OUTER_BOUND('',#5018,.T.);
#3675=FACE_OUTER_BOUND('',#5019,.T.);
#3676=FACE_OUTER_BOUND('',#5020,.T.);
#3677=FACE_OUTER_BOUND('',#5021,.T.);
#3678=FACE_OUTER_BOUND('',#5022,.T.);
#3679=FACE_OUTER_BOUND('',#5023,.T.);
#3680=FACE_OUTER_BOUND('',#5024,.T.);
#3681=FACE_OUTER_BOUND('',#5025,.T.);
#3682=FACE_OUTER_BOUND('',#5026,.T.);
#3683=FACE_OUTER_BOUND('',#5027,.T.);
#3684=FACE_OUTER_BOUND('',#5028,.T.);
#3685=FACE_OUTER_BOUND('',#5029,.T.);
#3686=FACE_OUTER_BOUND('',#5030,.T.);
#3687=FACE_OUTER_BOUND('',#5031,.T.);
#3688=FACE_OUTER_BOUND('',#5032,.T.);
#3689=FACE_OUTER_BOUND('',#5033,.T.);
#3690=FACE_OUTER_BOUND('',#5034,.T.);
#3691=FACE_OUTER_BOUND('',#5035,.T.);
#3692=FACE_OUTER_BOUND('',#5036,.T.);
#3693=FACE_OUTER_BOUND('',#5037,.T.);
#3694=FACE_OUTER_BOUND('',#5038,.T.);
#3695=FACE_OUTER_BOUND('',#5039,.T.);
#3696=FACE_OUTER_BOUND('',#5040,.T.);
#3697=FACE_OUTER_BOUND('',#5041,.T.);
#3698=FACE_OUTER_BOUND('',#5042,.T.);
#3699=FACE_OUTER_BOUND('',#5043,.T.);
#3700=FACE_OUTER_BOUND('',#5044,.T.);
#3701=FACE_OUTER_BOUND('',#5045,.T.);
#3702=FACE_OUTER_BOUND('',#5049,.T.);
#3703=FACE_OUTER_BOUND('',#5050,.T.);
#3704=FACE_OUTER_BOUND('',#5051,.T.);
#3705=FACE_OUTER_BOUND('',#5052,.T.);
#3706=FACE_OUTER_BOUND('',#5053,.T.);
#3707=FACE_OUTER_BOUND('',#5054,.T.);
#3708=FACE_OUTER_BOUND('',#5058,.T.);
#3709=FACE_OUTER_BOUND('',#5059,.T.);
#3710=FACE_OUTER_BOUND('',#5060,.T.);
#3711=FACE_OUTER_BOUND('',#5061,.T.);
#3712=FACE_OUTER_BOUND('',#5065,.T.);
#3713=FACE_OUTER_BOUND('',#5066,.T.);
#3714=FACE_OUTER_BOUND('',#5067,.T.);
#3715=FACE_OUTER_BOUND('',#5068,.T.);
#3716=FACE_OUTER_BOUND('',#5069,.T.);
#3717=FACE_OUTER_BOUND('',#5070,.T.);
#3718=FACE_OUTER_BOUND('',#5071,.T.);
#3719=FACE_OUTER_BOUND('',#5072,.T.);
#3720=FACE_OUTER_BOUND('',#5073,.T.);
#3721=FACE_OUTER_BOUND('',#5074,.T.);
#3722=FACE_OUTER_BOUND('',#5075,.T.);
#3723=FACE_OUTER_BOUND('',#5076,.T.);
#3724=FACE_OUTER_BOUND('',#5077,.T.);
#3725=FACE_OUTER_BOUND('',#5078,.T.);
#3726=FACE_OUTER_BOUND('',#5079,.T.);
#3727=FACE_OUTER_BOUND('',#5080,.T.);
#3728=FACE_OUTER_BOUND('',#5081,.T.);
#3729=FACE_OUTER_BOUND('',#5082,.T.);
#3730=FACE_OUTER_BOUND('',#5083,.T.);
#3731=FACE_OUTER_BOUND('',#5084,.T.);
#3732=FACE_OUTER_BOUND('',#5085,.T.);
#3733=FACE_OUTER_BOUND('',#5086,.T.);
#3734=FACE_OUTER_BOUND('',#5087,.T.);
#3735=FACE_OUTER_BOUND('',#5088,.T.);
#3736=FACE_OUTER_BOUND('',#5092,.T.);
#3737=FACE_OUTER_BOUND('',#5093,.T.);
#3738=FACE_OUTER_BOUND('',#5094,.T.);
#3739=FACE_OUTER_BOUND('',#5095,.T.);
#3740=FACE_OUTER_BOUND('',#5096,.T.);
#3741=FACE_OUTER_BOUND('',#5097,.T.);
#3742=FACE_OUTER_BOUND('',#5098,.T.);
#3743=FACE_OUTER_BOUND('',#5099,.T.);
#3744=FACE_OUTER_BOUND('',#5100,.T.);
#3745=FACE_OUTER_BOUND('',#5101,.T.);
#3746=FACE_OUTER_BOUND('',#5102,.T.);
#3747=FACE_OUTER_BOUND('',#5103,.T.);
#3748=FACE_OUTER_BOUND('',#5104,.T.);
#3749=FACE_OUTER_BOUND('',#5105,.T.);
#3750=FACE_OUTER_BOUND('',#5106,.T.);
#3751=FACE_OUTER_BOUND('',#5107,.T.);
#4943=EDGE_LOOP('',(#21633,#21634,#21635,#21636,#21637));
#4944=EDGE_LOOP('',(#21638));
#4945=EDGE_LOOP('',(#21639,#21640,#21641,#21642,#21643));
#4946=EDGE_LOOP('',(#21644));
#4947=EDGE_LOOP('',(#21645,#21646,#21647,#21648,#21649,#21650,#21651,#21652));
#4948=EDGE_LOOP('',(#21653,#21654));
#4949=EDGE_LOOP('',(#21655,#21656,#21657,#21658,#21659,#21660,#21661,#21662,
#21663,#21664,#21665,#21666,#21667,#21668,#21669,#21670,#21671,#21672,#21673,
#21674,#21675,#21676,#21677,#21678,#21679,#21680,#21681,#21682,#21683,#21684,
#21685,#21686,#21687,#21688,#21689,#21690,#21691,#21692,#21693,#21694,#21695,
#21696,#21697,#21698,#21699,#21700,#21701,#21702,#21703,#21704,#21705,#21706,
#21707,#21708,#21709,#21710,#21711,#21712,#21713,#21714,#21715,#21716));
#4950=EDGE_LOOP('',(#21717,#21718));
#4951=EDGE_LOOP('',(#21719,#21720,#21721,#21722,#21723,#21724,#21725,#21726,
#21727,#21728,#21729,#21730,#21731,#21732,#21733,#21734,#21735,#21736,#21737,
#21738,#21739,#21740,#21741,#21742,#21743,#21744,#21745,#21746,#21747,#21748,
#21749,#21750,#21751,#21752,#21753,#21754,#21755,#21756,#21757,#21758,#21759,
#21760,#21761,#21762,#21763,#21764,#21765,#21766,#21767,#21768,#21769,#21770,
#21771,#21772,#21773,#21774,#21775,#21776,#21777,#21778,#21779,#21780));
#4952=EDGE_LOOP('',(#21781,#21782));
#4953=EDGE_LOOP('',(#21783,#21784,#21785,#21786,#21787,#21788,#21789,#21790,
#21791,#21792,#21793,#21794,#21795,#21796,#21797,#21798,#21799,#21800,#21801,
#21802,#21803,#21804,#21805,#21806,#21807,#21808,#21809,#21810,#21811,#21812,
#21813,#21814,#21815,#21816,#21817,#21818,#21819,#21820,#21821,#21822,#21823,
#21824,#21825,#21826,#21827,#21828,#21829,#21830,#21831,#21832,#21833,#21834,
#21835,#21836,#21837,#21838,#21839,#21840,#21841,#21842,#21843,#21844));
#4954=EDGE_LOOP('',(#21845,#21846,#21847,#21848,#21849,#21850,#21851,#21852,
#21853,#21854));
#4955=EDGE_LOOP('',(#21855,#21856,#21857,#21858));
#4956=EDGE_LOOP('',(#21859,#21860,#21861,#21862));
#4957=EDGE_LOOP('',(#21863,#21864,#21865,#21866));
#4958=EDGE_LOOP('',(#21867,#21868,#21869,#21870));
#4959=EDGE_LOOP('',(#21871,#21872,#21873,#21874));
#4960=EDGE_LOOP('',(#21875,#21876,#21877,#21878));
#4961=EDGE_LOOP('',(#21879,#21880,#21881,#21882));
#4962=EDGE_LOOP('',(#21883,#21884,#21885,#21886));
#4963=EDGE_LOOP('',(#21887,#21888,#21889,#21890));
#4964=EDGE_LOOP('',(#21891,#21892,#21893,#21894,#21895));
#4965=EDGE_LOOP('',(#21896,#21897,#21898,#21899));
#4966=EDGE_LOOP('',(#21900,#21901,#21902,#21903,#21904));
#4967=EDGE_LOOP('',(#21905,#21906,#21907,#21908));
#4968=EDGE_LOOP('',(#21909,#21910,#21911,#21912));
#4969=EDGE_LOOP('',(#21913,#21914,#21915,#21916));
#4970=EDGE_LOOP('',(#21917,#21918,#21919,#21920));
#4971=EDGE_LOOP('',(#21921,#21922,#21923,#21924));
#4972=EDGE_LOOP('',(#21925,#21926,#21927,#21928));
#4973=EDGE_LOOP('',(#21929,#21930,#21931,#21932));
#4974=EDGE_LOOP('',(#21933,#21934,#21935,#21936));
#4975=EDGE_LOOP('',(#21937,#21938,#21939,#21940));
#4976=EDGE_LOOP('',(#21941,#21942,#21943,#21944));
#4977=EDGE_LOOP('',(#21945,#21946,#21947,#21948));
#4978=EDGE_LOOP('',(#21949,#21950,#21951,#21952));
#4979=EDGE_LOOP('',(#21953,#21954,#21955,#21956,#21957));
#4980=EDGE_LOOP('',(#21958,#21959,#21960,#21961));
#4981=EDGE_LOOP('',(#21962,#21963,#21964,#21965,#21966));
#4982=EDGE_LOOP('',(#21967,#21968,#21969,#21970));
#4983=EDGE_LOOP('',(#21971,#21972,#21973,#21974));
#4984=EDGE_LOOP('',(#21975,#21976,#21977,#21978));
#4985=EDGE_LOOP('',(#21979,#21980,#21981,#21982));
#4986=EDGE_LOOP('',(#21983,#21984,#21985,#21986));
#4987=EDGE_LOOP('',(#21987,#21988,#21989,#21990));
#4988=EDGE_LOOP('',(#21991,#21992,#21993,#21994,#21995,#21996,#21997,#21998,
#21999,#22000));
#4989=EDGE_LOOP('',(#22001,#22002,#22003,#22004));
#4990=EDGE_LOOP('',(#22005,#22006,#22007,#22008));
#4991=EDGE_LOOP('',(#22009,#22010,#22011,#22012));
#4992=EDGE_LOOP('',(#22013,#22014,#22015,#22016));
#4993=EDGE_LOOP('',(#22017,#22018,#22019,#22020));
#4994=EDGE_LOOP('',(#22021,#22022,#22023,#22024));
#4995=EDGE_LOOP('',(#22025,#22026,#22027,#22028));
#4996=EDGE_LOOP('',(#22029,#22030,#22031,#22032));
#4997=EDGE_LOOP('',(#22033,#22034,#22035,#22036));
#4998=EDGE_LOOP('',(#22037,#22038,#22039,#22040));
#4999=EDGE_LOOP('',(#22041,#22042,#22043,#22044,#22045));
#5000=EDGE_LOOP('',(#22046,#22047,#22048,#22049,#22050));
#5001=EDGE_LOOP('',(#22051,#22052,#22053,#22054));
#5002=EDGE_LOOP('',(#22055,#22056,#22057,#22058));
#5003=EDGE_LOOP('',(#22059,#22060,#22061,#22062));
#5004=EDGE_LOOP('',(#22063,#22064,#22065,#22066));
#5005=EDGE_LOOP('',(#22067,#22068,#22069,#22070));
#5006=EDGE_LOOP('',(#22071,#22072,#22073,#22074));
#5007=EDGE_LOOP('',(#22075,#22076,#22077,#22078));
#5008=EDGE_LOOP('',(#22079,#22080,#22081,#22082));
#5009=EDGE_LOOP('',(#22083,#22084,#22085,#22086));
#5010=EDGE_LOOP('',(#22087,#22088,#22089,#22090));
#5011=EDGE_LOOP('',(#22091,#22092,#22093,#22094));
#5012=EDGE_LOOP('',(#22095,#22096,#22097,#22098));
#5013=EDGE_LOOP('',(#22099,#22100,#22101,#22102));
#5014=EDGE_LOOP('',(#22103,#22104,#22105,#22106,#22107));
#5015=EDGE_LOOP('',(#22108,#22109,#22110,#22111,#22112));
#5016=EDGE_LOOP('',(#22113,#22114,#22115,#22116));
#5017=EDGE_LOOP('',(#22117,#22118,#22119,#22120));
#5018=EDGE_LOOP('',(#22121,#22122,#22123,#22124));
#5019=EDGE_LOOP('',(#22125,#22126,#22127,#22128));
#5020=EDGE_LOOP('',(#22129,#22130,#22131,#22132));
#5021=EDGE_LOOP('',(#22133,#22134,#22135,#22136));
#5022=EDGE_LOOP('',(#22137,#22138,#22139,#22140));
#5023=EDGE_LOOP('',(#22141,#22142,#22143,#22144));
#5024=EDGE_LOOP('',(#22145,#22146,#22147,#22148));
#5025=EDGE_LOOP('',(#22149,#22150,#22151,#22152));
#5026=EDGE_LOOP('',(#22153,#22154,#22155,#22156,#22157,#22158,#22159,#22160));
#5027=EDGE_LOOP('',(#22161,#22162,#22163,#22164));
#5028=EDGE_LOOP('',(#22165,#22166,#22167,#22168));
#5029=EDGE_LOOP('',(#22169,#22170,#22171,#22172,#22173,#22174,#22175,#22176,
#22177,#22178));
#5030=EDGE_LOOP('',(#22179,#22180,#22181,#22182));
#5031=EDGE_LOOP('',(#22183,#22184,#22185,#22186));
#5032=EDGE_LOOP('',(#22187,#22188,#22189,#22190,#22191));
#5033=EDGE_LOOP('',(#22192,#22193,#22194,#22195));
#5034=EDGE_LOOP('',(#22196,#22197,#22198,#22199));
#5035=EDGE_LOOP('',(#22200,#22201,#22202,#22203));
#5036=EDGE_LOOP('',(#22204,#22205,#22206,#22207));
#5037=EDGE_LOOP('',(#22208,#22209,#22210,#22211,#22212));
#5038=EDGE_LOOP('',(#22213,#22214,#22215,#22216));
#5039=EDGE_LOOP('',(#22217,#22218,#22219,#22220));
#5040=EDGE_LOOP('',(#22221,#22222,#22223,#22224));
#5041=EDGE_LOOP('',(#22225,#22226,#22227,#22228));
#5042=EDGE_LOOP('',(#22229,#22230,#22231,#22232));
#5043=EDGE_LOOP('',(#22233,#22234,#22235,#22236));
#5044=EDGE_LOOP('',(#22237,#22238,#22239,#22240));
#5045=EDGE_LOOP('',(#22241,#22242,#22243,#22244));
#5046=EDGE_LOOP('',(#22245));
#5047=EDGE_LOOP('',(#22246));
#5048=EDGE_LOOP('',(#22247));
#5049=EDGE_LOOP('',(#22248,#22249,#22250,#22251));
#5050=EDGE_LOOP('',(#22252,#22253,#22254,#22255));
#5051=EDGE_LOOP('',(#22256,#22257,#22258,#22259));
#5052=EDGE_LOOP('',(#22260,#22261,#22262,#22263));
#5053=EDGE_LOOP('',(#22264,#22265,#22266,#22267));
#5054=EDGE_LOOP('',(#22268,#22269,#22270,#22271));
#5055=EDGE_LOOP('',(#22272));
#5056=EDGE_LOOP('',(#22273));
#5057=EDGE_LOOP('',(#22274));
#5058=EDGE_LOOP('',(#22275,#22276,#22277,#22278));
#5059=EDGE_LOOP('',(#22279,#22280,#22281,#22282));
#5060=EDGE_LOOP('',(#22283,#22284,#22285,#22286));
#5061=EDGE_LOOP('',(#22287,#22288,#22289,#22290));
#5062=EDGE_LOOP('',(#22291));
#5063=EDGE_LOOP('',(#22292));
#5064=EDGE_LOOP('',(#22293));
#5065=EDGE_LOOP('',(#22294,#22295,#22296,#22297));
#5066=EDGE_LOOP('',(#22298,#22299,#22300,#22301));
#5067=EDGE_LOOP('',(#22302,#22303,#22304,#22305));
#5068=EDGE_LOOP('',(#22306,#22307,#22308,#22309));
#5069=EDGE_LOOP('',(#22310,#22311,#22312,#22313));
#5070=EDGE_LOOP('',(#22314,#22315,#22316,#22317));
#5071=EDGE_LOOP('',(#22318,#22319,#22320,#22321));
#5072=EDGE_LOOP('',(#22322,#22323,#22324,#22325,#22326,#22327,#22328,#22329,
#22330,#22331));
#5073=EDGE_LOOP('',(#22332,#22333,#22334,#22335));
#5074=EDGE_LOOP('',(#22336,#22337,#22338,#22339));
#5075=EDGE_LOOP('',(#22340,#22341,#22342,#22343,#22344));
#5076=EDGE_LOOP('',(#22345,#22346,#22347,#22348));
#5077=EDGE_LOOP('',(#22349,#22350,#22351,#22352));
#5078=EDGE_LOOP('',(#22353,#22354,#22355,#22356));
#5079=EDGE_LOOP('',(#22357,#22358,#22359,#22360));
#5080=EDGE_LOOP('',(#22361,#22362,#22363,#22364,#22365));
#5081=EDGE_LOOP('',(#22366,#22367,#22368,#22369));
#5082=EDGE_LOOP('',(#22370,#22371,#22372,#22373));
#5083=EDGE_LOOP('',(#22374,#22375,#22376,#22377));
#5084=EDGE_LOOP('',(#22378,#22379,#22380,#22381));
#5085=EDGE_LOOP('',(#22382,#22383,#22384,#22385));
#5086=EDGE_LOOP('',(#22386,#22387,#22388,#22389));
#5087=EDGE_LOOP('',(#22390,#22391,#22392,#22393));
#5088=EDGE_LOOP('',(#22394,#22395,#22396,#22397));
#5089=EDGE_LOOP('',(#22398,#22399,#22400));
#5090=EDGE_LOOP('',(#22401,#22402,#22403));
#5091=EDGE_LOOP('',(#22404,#22405,#22406));
#5092=EDGE_LOOP('',(#22407,#22408,#22409,#22410));
#5093=EDGE_LOOP('',(#22411,#22412,#22413,#22414));
#5094=EDGE_LOOP('',(#22415,#22416,#22417,#22418));
#5095=EDGE_LOOP('',(#22419,#22420,#22421,#22422));
#5096=EDGE_LOOP('',(#22423,#22424,#22425,#22426));
#5097=EDGE_LOOP('',(#22427,#22428,#22429,#22430));
#5098=EDGE_LOOP('',(#22431,#22432,#22433,#22434));
#5099=EDGE_LOOP('',(#22435,#22436,#22437,#22438));
#5100=EDGE_LOOP('',(#22439,#22440,#22441,#22442));
#5101=EDGE_LOOP('',(#22443,#22444,#22445,#22446));
#5102=EDGE_LOOP('',(#22447,#22448,#22449,#22450));
#5103=EDGE_LOOP('',(#22451,#22452,#22453,#22454));
#5104=EDGE_LOOP('',(#22455,#22456,#22457,#22458));
#5105=EDGE_LOOP('',(#22459,#22460,#22461,#22462));
#5106=EDGE_LOOP('',(#22463,#22464,#22465,#22466,#22467,#22468,#22469,#22470,
#22471,#22472,#22473,#22474,#22475,#22476,#22477,#22478,#22479,#22480,#22481,
#22482,#22483,#22484,#22485,#22486,#22487,#22488,#22489,#22490,#22491,#22492,
#22493,#22494,#22495,#22496,#22497,#22498,#22499,#22500,#22501,#22502,#22503,
#22504,#22505,#22506,#22507,#22508,#22509,#22510,#22511,#22512,#22513,#22514,
#22515,#22516,#22517,#22518,#22519,#22520,#22521,#22522,#22523,#22524,#22525,
#22526,#22527,#22528,#22529,#22530,#22531,#22532,#22533,#22534));
#5107=EDGE_LOOP('',(#22535,#22536,#22537,#22538,#22539,#22540,#22541,#22542,
#22543,#22544,#22545,#22546,#22547,#22548,#22549,#22550,#22551,#22552,#22553,
#22554,#22555,#22556,#22557,#22558,#22559,#22560,#22561,#22562,#22563,#22564,
#22565,#22566,#22567,#22568,#22569,#22570,#22571,#22572,#22573,#22574,#22575,
#22576,#22577,#22578,#22579,#22580,#22581,#22582,#22583,#22584,#22585,#22586,
#22587,#22588,#22589,#22590,#22591,#22592,#22593,#22594,#22595,#22596,#22597,
#22598,#22599,#22600,#22601,#22602,#22603,#22604,#22605,#22606));
#5992=CIRCLE('',#29153,3.00000000191135);
#5993=CIRCLE('',#29154,3.);
#5994=CIRCLE('',#29155,3.);
#5995=CIRCLE('',#29158,3.00000000191136);
#5996=CIRCLE('',#29159,3.00000000000001);
#5997=CIRCLE('',#29160,3.00000000000001);
#5998=CIRCLE('',#29164,3.);
#5999=CIRCLE('',#29166,3.);
#6000=CIRCLE('',#29167,3.);
#6001=CIRCLE('',#29168,3.);
#6002=CIRCLE('',#29175,3.00000000191135);
#6003=CIRCLE('',#29176,3.00000000191135);
#6004=CIRCLE('',#29177,3.00000000191135);
#6005=CIRCLE('',#29178,3.00000000191135);
#6006=CIRCLE('',#29184,3.);
#6007=CIRCLE('',#29186,3.);
#6008=CIRCLE('',#29187,3.);
#6009=CIRCLE('',#29188,3.);
#6010=CIRCLE('',#29195,3.00000000191135);
#6011=CIRCLE('',#29196,3.00000000191135);
#6012=CIRCLE('',#29197,3.00000000191135);
#6013=CIRCLE('',#29198,3.00000000191135);
#6014=CIRCLE('',#29204,3.00000000000001);
#6015=CIRCLE('',#29206,3.00000000000001);
#6016=CIRCLE('',#29207,3.00000000000001);
#6017=CIRCLE('',#29208,3.00000000000001);
#6018=CIRCLE('',#29215,3.00000000191136);
#6019=CIRCLE('',#29216,3.00000000191136);
#6020=CIRCLE('',#29217,3.00000000191136);
#6021=CIRCLE('',#29218,3.00000000191136);
#6022=CIRCLE('',#29224,0.3);
#6023=CIRCLE('',#29225,0.3);
#6024=CIRCLE('',#29230,0.499999999999998);
#6025=CIRCLE('',#29232,0.499999999999998);
#6026=CIRCLE('',#29238,1.);
#6027=CIRCLE('',#29240,1.);
#6028=CIRCLE('',#29246,2.);
#6029=CIRCLE('',#29248,2.);
#6030=CIRCLE('',#29254,5.);
#6031=CIRCLE('',#29256,5.);
#6032=CIRCLE('',#29262,0.800000000000001);
#6033=CIRCLE('',#29264,0.800000000000001);
#6034=CIRCLE('',#29270,0.3);
#6035=CIRCLE('',#29271,0.3);
#6036=CIRCLE('',#29276,0.499999999999998);
#6037=CIRCLE('',#29283,1.);
#6038=CIRCLE('',#29290,2.);
#6039=CIRCLE('',#29297,5.);
#6040=CIRCLE('',#29304,0.800000000000001);
#6041=CIRCLE('',#29311,2.5);
#6042=CIRCLE('',#29312,2.5);
#6043=CIRCLE('',#29314,2.5);
#6044=CIRCLE('',#29315,2.5);
#6045=CIRCLE('',#29317,2.5);
#6046=CIRCLE('',#29318,2.5);
#6047=CIRCLE('',#29322,0.3);
#6048=CIRCLE('',#29323,0.3);
#6049=CIRCLE('',#29326,0.300000000000002);
#6050=CIRCLE('',#29327,0.300000000000002);
#6051=CIRCLE('',#29341,0.300000000000002);
#6052=CIRCLE('',#29342,0.300000000000002);
#6053=CIRCLE('',#29345,0.500000000000001);
#6054=CIRCLE('',#29346,0.500000000000001);
#6055=CIRCLE('',#29349,0.508000000000002);
#6056=CIRCLE('',#29350,0.508000000000002);
#6057=CIRCLE('',#29353,3.);
#6058=CIRCLE('',#29354,3.);
#6059=CIRCLE('',#29357,5.);
#6060=CIRCLE('',#29358,5.);
#6061=CIRCLE('',#29361,1.);
#6062=CIRCLE('',#29362,1.);
#6063=CIRCLE('',#29367,1.);
#6064=CIRCLE('',#29368,1.);
#6065=CIRCLE('',#29374,0.3);
#6066=CIRCLE('',#29375,0.3);
#6067=CIRCLE('',#29378,0.300000000000002);
#6068=CIRCLE('',#29379,0.300000000000002);
#6069=CIRCLE('',#29382,0.800000000000001);
#6070=CIRCLE('',#29385,5.);
#6071=CIRCLE('',#29388,2.);
#6072=CIRCLE('',#29391,1.);
#6073=CIRCLE('',#29394,0.499999999999998);
#6074=CIRCLE('',#29398,0.300000000000002);
#6075=CIRCLE('',#29399,0.300000000000002);
#6076=CIRCLE('',#29402,0.5);
#6077=CIRCLE('',#29403,0.5);
#6078=CIRCLE('',#29406,0.508000000000002);
#6079=CIRCLE('',#29407,0.508000000000002);
#6080=CIRCLE('',#29410,3.);
#6081=CIRCLE('',#29411,3.);
#6082=CIRCLE('',#29414,5.);
#6083=CIRCLE('',#29415,5.);
#6084=CIRCLE('',#29418,1.);
#6085=CIRCLE('',#29419,1.);
#6086=CIRCLE('',#29424,1.);
#6087=CIRCLE('',#29425,1.);
#7088=LINE('',#125624,#8933);
#7089=LINE('',#125633,#8934);
#7090=LINE('',#125637,#8935);
#7091=LINE('',#125639,#8936);
#7092=LINE('',#125641,#8937);
#7093=LINE('',#125643,#8938);
#7094=LINE('',#125645,#8939);
#7095=LINE('',#125646,#8940);
#7096=LINE('',#125650,#8941);
#7097=LINE('',#125656,#8942);
#7098=LINE('',#125676,#8943);
#7099=LINE('',#125705,#8944);
#7100=LINE('',#125736,#8945);
#7101=LINE('',#125764,#8946);
#7102=LINE('',#125793,#8947);
#7103=LINE('',#125814,#8948);
#7104=LINE('',#125835,#8949);
#7105=LINE('',#125864,#8950);
#7106=LINE('',#125894,#8951);
#7107=LINE('',#125933,#8952);
#7108=LINE('',#125967,#8953);
#7109=LINE('',#125993,#8954);
#7110=LINE('',#126015,#8955);
#7111=LINE('',#126037,#8956);
#7112=LINE('',#126056,#8957);
#7113=LINE('',#126062,#8958);
#7114=LINE('',#126082,#8959);
#7115=LINE('',#126111,#8960);
#7116=LINE('',#126142,#8961);
#7117=LINE('',#126170,#8962);
#7118=LINE('',#126199,#8963);
#7119=LINE('',#126220,#8964);
#7120=LINE('',#126241,#8965);
#7121=LINE('',#126270,#8966);
#7122=LINE('',#126300,#8967);
#7123=LINE('',#126339,#8968);
#7124=LINE('',#126373,#8969);
#7125=LINE('',#126399,#8970);
#7126=LINE('',#126421,#8971);
#7127=LINE('',#126443,#8972);
#7128=LINE('',#126462,#8973);
#7129=LINE('',#126468,#8974);
#7130=LINE('',#126490,#8975);
#7131=LINE('',#126519,#8976);
#7132=LINE('',#126552,#8977);
#7133=LINE('',#126580,#8978);
#7134=LINE('',#126609,#8979);
#7135=LINE('',#126630,#8980);
#7136=LINE('',#126651,#8981);
#7137=LINE('',#126680,#8982);
#7138=LINE('',#126710,#8983);
#7139=LINE('',#126749,#8984);
#7140=LINE('',#126783,#8985);
#7141=LINE('',#126809,#8986);
#7142=LINE('',#126831,#8987);
#7143=LINE('',#126853,#8988);
#7144=LINE('',#126871,#8989);
#7145=LINE('',#126875,#8990);
#7146=LINE('',#126878,#8991);
#7147=LINE('',#126879,#8992);
#7148=LINE('',#126880,#8993);
#7149=LINE('',#126883,#8994);
#7150=LINE('',#126884,#8995);
#7151=LINE('',#126887,#8996);
#7152=LINE('',#126888,#8997);
#7153=LINE('',#126890,#8998);
#7154=LINE('',#126893,#8999);
#7155=LINE('',#126898,#9000);
#7156=LINE('',#126900,#9001);
#7157=LINE('',#126903,#9002);
#7158=LINE('',#126904,#9003);
#7159=LINE('',#126907,#9004);
#7160=LINE('',#126908,#9005);
#7161=LINE('',#126910,#9006);
#7162=LINE('',#126913,#9007);
#7163=LINE('',#126918,#9008);
#7164=LINE('',#126920,#9009);
#7165=LINE('',#126923,#9010);
#7166=LINE('',#126924,#9011);
#7167=LINE('',#126927,#9012);
#7168=LINE('',#126928,#9013);
#7169=LINE('',#126930,#9014);
#7170=LINE('',#126933,#9015);
#7171=LINE('',#126938,#9016);
#7172=LINE('',#126940,#9017);
#7173=LINE('',#126943,#9018);
#7174=LINE('',#126944,#9019);
#7175=LINE('',#126947,#9020);
#7176=LINE('',#126948,#9021);
#7177=LINE('',#126950,#9022);
#7178=LINE('',#126953,#9023);
#7179=LINE('',#126958,#9024);
#7180=LINE('',#126960,#9025);
#7181=LINE('',#126963,#9026);
#7182=LINE('',#126964,#9027);
#7183=LINE('',#126967,#9028);
#7184=LINE('',#126968,#9029);
#7185=LINE('',#126970,#9030);
#7186=LINE('',#126973,#9031);
#7187=LINE('',#126978,#9032);
#7188=LINE('',#126980,#9033);
#7189=LINE('',#126983,#9034);
#7190=LINE('',#126984,#9035);
#7191=LINE('',#126987,#9036);
#7192=LINE('',#126988,#9037);
#7193=LINE('',#126990,#9038);
#7194=LINE('',#126992,#9039);
#7195=LINE('',#126993,#9040);
#7196=LINE('',#126995,#9041);
#7197=LINE('',#126999,#9042);
#7198=LINE('',#127002,#9043);
#7199=LINE('',#127005,#9044);
#7200=LINE('',#127006,#9045);
#7201=LINE('',#127008,#9046);
#7202=LINE('',#127010,#9047);
#7203=LINE('',#127013,#9048);
#7204=LINE('',#127016,#9049);
#7205=LINE('',#127018,#9050);
#7206=LINE('',#127021,#9051);
#7207=LINE('',#127022,#9052);
#7208=LINE('',#127024,#9053);
#7209=LINE('',#127026,#9054);
#7210=LINE('',#127029,#9055);
#7211=LINE('',#127032,#9056);
#7212=LINE('',#127034,#9057);
#7213=LINE('',#127037,#9058);
#7214=LINE('',#127038,#9059);
#7215=LINE('',#127040,#9060);
#7216=LINE('',#127042,#9061);
#7217=LINE('',#127045,#9062);
#7218=LINE('',#127048,#9063);
#7219=LINE('',#127050,#9064);
#7220=LINE('',#127053,#9065);
#7221=LINE('',#127054,#9066);
#7222=LINE('',#127056,#9067);
#7223=LINE('',#127058,#9068);
#7224=LINE('',#127061,#9069);
#7225=LINE('',#127064,#9070);
#7226=LINE('',#127066,#9071);
#7227=LINE('',#127069,#9072);
#7228=LINE('',#127070,#9073);
#7229=LINE('',#127072,#9074);
#7230=LINE('',#127074,#9075);
#7231=LINE('',#127077,#9076);
#7232=LINE('',#127080,#9077);
#7233=LINE('',#127082,#9078);
#7234=LINE('',#127085,#9079);
#7235=LINE('',#127086,#9080);
#7236=LINE('',#127088,#9081);
#7237=LINE('',#127090,#9082);
#7238=LINE('',#127095,#9083);
#7239=LINE('',#127101,#9084);
#7240=LINE('',#127107,#9085);
#7241=LINE('',#127112,#9086);
#7242=LINE('',#127114,#9087);
#7243=LINE('',#127116,#9088);
#7244=LINE('',#127117,#9089);
#7245=LINE('',#127120,#9090);
#7246=LINE('',#127122,#9091);
#7247=LINE('',#127123,#9092);
#7248=LINE('',#127128,#9093);
#7249=LINE('',#127132,#9094);
#7250=LINE('',#127134,#9095);
#7251=LINE('',#127135,#9096);
#7252=LINE('',#127137,#9097);
#7253=LINE('',#127141,#9098);
#7254=LINE('',#127143,#9099);
#7255=LINE('',#127145,#9100);
#7256=LINE('',#127147,#9101);
#7257=LINE('',#127149,#9102);
#7258=LINE('',#127151,#9103);
#7259=LINE('',#127153,#9104);
#7260=LINE('',#127155,#9105);
#7261=LINE('',#127157,#9106);
#7262=LINE('',#127159,#9107);
#7263=LINE('',#127163,#9108);
#7264=LINE('',#127165,#9109);
#7265=LINE('',#127166,#9110);
#7266=LINE('',#127171,#9111);
#7267=LINE('',#127175,#9112);
#7268=LINE('',#127177,#9113);
#7269=LINE('',#127178,#9114);
#7270=LINE('',#127183,#9115);
#7271=LINE('',#127187,#9116);
#7272=LINE('',#127189,#9117);
#7273=LINE('',#127190,#9118);
#7274=LINE('',#127195,#9119);
#7275=LINE('',#127199,#9120);
#7276=LINE('',#127201,#9121);
#7277=LINE('',#127202,#9122);
#7278=LINE('',#127207,#9123);
#7279=LINE('',#127211,#9124);
#7280=LINE('',#127213,#9125);
#7281=LINE('',#127214,#9126);
#7282=LINE('',#127219,#9127);
#7283=LINE('',#127223,#9128);
#7284=LINE('',#127225,#9129);
#7285=LINE('',#127226,#9130);
#7286=LINE('',#127231,#9131);
#7287=LINE('',#127235,#9132);
#7288=LINE('',#127237,#9133);
#7289=LINE('',#127238,#9134);
#7290=LINE('',#127241,#9135);
#7291=LINE('',#127243,#9136);
#7292=LINE('',#127244,#9137);
#7293=LINE('',#127247,#9138);
#7294=LINE('',#127249,#9139);
#7295=LINE('',#127250,#9140);
#7296=LINE('',#127255,#9141);
#7297=LINE('',#127259,#9142);
#7298=LINE('',#127261,#9143);
#7299=LINE('',#127262,#9144);
#7300=LINE('',#127265,#9145);
#7301=LINE('',#127267,#9146);
#7302=LINE('',#127268,#9147);
#7303=LINE('',#127270,#9148);
#7304=LINE('',#127271,#9149);
#7305=LINE('',#127274,#9150);
#7306=LINE('',#127276,#9151);
#7307=LINE('',#127277,#9152);
#7308=LINE('',#127283,#9153);
#7309=LINE('',#127286,#9154);
#7310=LINE('',#127288,#9155);
#7311=LINE('',#127289,#9156);
#7312=LINE('',#127292,#9157);
#7313=LINE('',#127297,#9158);
#7314=LINE('',#127298,#9159);
#7315=LINE('',#127301,#9160);
#7316=LINE('',#127305,#9161);
#7317=LINE('',#127306,#9162);
#7318=LINE('',#127309,#9163);
#7319=LINE('',#127313,#9164);
#7320=LINE('',#127314,#9165);
#7321=LINE('',#127317,#9166);
#7322=LINE('',#127321,#9167);
#7323=LINE('',#127322,#9168);
#7324=LINE('',#127325,#9169);
#7325=LINE('',#127329,#9170);
#7326=LINE('',#127330,#9171);
#7327=LINE('',#127333,#9172);
#7328=LINE('',#127336,#9173);
#7329=LINE('',#127339,#9174);
#7330=LINE('',#127341,#9175);
#7331=LINE('',#127342,#9176);
#7332=LINE('',#127348,#9177);
#7333=LINE('',#127351,#9178);
#7334=LINE('',#127353,#9179);
#7335=LINE('',#127354,#9180);
#7336=LINE('',#127360,#9181);
#7337=LINE('',#127363,#9182);
#7338=LINE('',#127365,#9183);
#7339=LINE('',#127366,#9184);
#7340=LINE('',#127372,#9185);
#7341=LINE('',#127375,#9186);
#7342=LINE('',#127377,#9187);
#7343=LINE('',#127378,#9188);
#7344=LINE('',#127384,#9189);
#7345=LINE('',#127387,#9190);
#7346=LINE('',#127389,#9191);
#7347=LINE('',#127390,#9192);
#7348=LINE('',#127396,#9193);
#7349=LINE('',#127399,#9194);
#7350=LINE('',#127401,#9195);
#7351=LINE('',#127402,#9196);
#7352=LINE('',#127408,#9197);
#7353=LINE('',#127411,#9198);
#7354=LINE('',#127413,#9199);
#7355=LINE('',#127414,#9200);
#7356=LINE('',#127417,#9201);
#7357=LINE('',#127419,#9202);
#7358=LINE('',#127420,#9203);
#7359=LINE('',#127423,#9204);
#7360=LINE('',#127425,#9205);
#7361=LINE('',#127426,#9206);
#7362=LINE('',#127432,#9207);
#7363=LINE('',#127435,#9208);
#7364=LINE('',#127437,#9209);
#7365=LINE('',#127438,#9210);
#7366=LINE('',#127441,#9211);
#7367=LINE('',#127443,#9212);
#7368=LINE('',#127444,#9213);
#7369=LINE('',#127446,#9214);
#7370=LINE('',#127447,#9215);
#8933=VECTOR('',#32910,3.);
#8934=VECTOR('',#32921,3.00000000000001);
#8935=VECTOR('',#32928,10.);
#8936=VECTOR('',#32929,10.);
#8937=VECTOR('',#32930,10.);
#8938=VECTOR('',#32931,10.);
#8939=VECTOR('',#32932,10.);
#8940=VECTOR('',#32933,10.);
#8941=VECTOR('',#32936,10.);
#8942=VECTOR('',#32943,3.);
#8943=VECTOR('',#32946,10.);
#8944=VECTOR('',#32947,10.);
#8945=VECTOR('',#32952,10.);
#8946=VECTOR('',#32955,10.);
#8947=VECTOR('',#32956,10.);
#8948=VECTOR('',#32959,3.);
#8949=VECTOR('',#32962,10.);
#8950=VECTOR('',#32963,10.);
#8951=VECTOR('',#32966,10.);
#8952=VECTOR('',#32971,10.);
#8953=VECTOR('',#32972,10.);
#8954=VECTOR('',#32975,3.);
#8955=VECTOR('',#32982,10.);
#8956=VECTOR('',#32987,10.);
#8957=VECTOR('',#32992,10.);
#8958=VECTOR('',#32999,3.);
#8959=VECTOR('',#33002,10.);
#8960=VECTOR('',#33003,10.);
#8961=VECTOR('',#33008,10.);
#8962=VECTOR('',#33011,10.);
#8963=VECTOR('',#33012,10.);
#8964=VECTOR('',#33015,3.);
#8965=VECTOR('',#33018,10.);
#8966=VECTOR('',#33019,10.);
#8967=VECTOR('',#33022,10.);
#8968=VECTOR('',#33027,10.);
#8969=VECTOR('',#33028,10.);
#8970=VECTOR('',#33031,3.);
#8971=VECTOR('',#33038,10.);
#8972=VECTOR('',#33043,10.);
#8973=VECTOR('',#33048,10.);
#8974=VECTOR('',#33055,3.00000000000001);
#8975=VECTOR('',#33058,10.);
#8976=VECTOR('',#33059,10.);
#8977=VECTOR('',#33064,10.);
#8978=VECTOR('',#33067,10.);
#8979=VECTOR('',#33068,10.);
#8980=VECTOR('',#33071,3.00000000000001);
#8981=VECTOR('',#33074,10.);
#8982=VECTOR('',#33075,10.);
#8983=VECTOR('',#33078,10.);
#8984=VECTOR('',#33083,10.);
#8985=VECTOR('',#33084,10.);
#8986=VECTOR('',#33087,3.00000000000001);
#8987=VECTOR('',#33094,10.);
#8988=VECTOR('',#33099,10.);
#8989=VECTOR('',#33104,10.);
#8990=VECTOR('',#33107,10.);
#8991=VECTOR('',#33110,10.);
#8992=VECTOR('',#33111,10.);
#8993=VECTOR('',#33112,10.);
#8994=VECTOR('',#33115,10.);
#8995=VECTOR('',#33116,10.);
#8996=VECTOR('',#33119,10.);
#8997=VECTOR('',#33120,10.);
#8998=VECTOR('',#33123,10.);
#8999=VECTOR('',#33126,10.);
#9000=VECTOR('',#33133,10.);
#9001=VECTOR('',#33136,10.);
#9002=VECTOR('',#33139,10.);
#9003=VECTOR('',#33140,10.);
#9004=VECTOR('',#33143,10.);
#9005=VECTOR('',#33144,10.);
#9006=VECTOR('',#33147,10.);
#9007=VECTOR('',#33150,10.);
#9008=VECTOR('',#33157,10.);
#9009=VECTOR('',#33160,10.);
#9010=VECTOR('',#33163,10.);
#9011=VECTOR('',#33164,10.);
#9012=VECTOR('',#33167,10.);
#9013=VECTOR('',#33168,10.);
#9014=VECTOR('',#33171,10.);
#9015=VECTOR('',#33174,10.);
#9016=VECTOR('',#33181,10.);
#9017=VECTOR('',#33184,10.);
#9018=VECTOR('',#33187,10.);
#9019=VECTOR('',#33188,10.);
#9020=VECTOR('',#33191,10.);
#9021=VECTOR('',#33192,10.);
#9022=VECTOR('',#33195,10.);
#9023=VECTOR('',#33198,10.);
#9024=VECTOR('',#33205,10.);
#9025=VECTOR('',#33208,10.);
#9026=VECTOR('',#33211,10.);
#9027=VECTOR('',#33212,10.);
#9028=VECTOR('',#33215,10.);
#9029=VECTOR('',#33216,10.);
#9030=VECTOR('',#33219,10.);
#9031=VECTOR('',#33222,10.);
#9032=VECTOR('',#33229,10.);
#9033=VECTOR('',#33232,10.);
#9034=VECTOR('',#33235,10.);
#9035=VECTOR('',#33236,10.);
#9036=VECTOR('',#33239,10.);
#9037=VECTOR('',#33240,10.);
#9038=VECTOR('',#33243,10.);
#9039=VECTOR('',#33246,10.);
#9040=VECTOR('',#33247,10.);
#9041=VECTOR('',#33248,10.);
#9042=VECTOR('',#33251,10.);
#9043=VECTOR('',#33254,10.);
#9044=VECTOR('',#33257,10.);
#9045=VECTOR('',#33258,10.);
#9046=VECTOR('',#33261,10.);
#9047=VECTOR('',#33264,10.);
#9048=VECTOR('',#33267,10.);
#9049=VECTOR('',#33272,10.);
#9050=VECTOR('',#33275,10.);
#9051=VECTOR('',#33278,10.);
#9052=VECTOR('',#33279,10.);
#9053=VECTOR('',#33282,10.);
#9054=VECTOR('',#33285,10.);
#9055=VECTOR('',#33288,10.);
#9056=VECTOR('',#33293,10.);
#9057=VECTOR('',#33296,10.);
#9058=VECTOR('',#33299,10.);
#9059=VECTOR('',#33300,10.);
#9060=VECTOR('',#33303,10.);
#9061=VECTOR('',#33306,10.);
#9062=VECTOR('',#33309,10.);
#9063=VECTOR('',#33314,10.);
#9064=VECTOR('',#33317,10.);
#9065=VECTOR('',#33320,10.);
#9066=VECTOR('',#33321,10.);
#9067=VECTOR('',#33324,10.);
#9068=VECTOR('',#33327,10.);
#9069=VECTOR('',#33330,10.);
#9070=VECTOR('',#33335,10.);
#9071=VECTOR('',#33338,10.);
#9072=VECTOR('',#33341,10.);
#9073=VECTOR('',#33342,10.);
#9074=VECTOR('',#33345,10.);
#9075=VECTOR('',#33348,10.);
#9076=VECTOR('',#33351,10.);
#9077=VECTOR('',#33356,10.);
#9078=VECTOR('',#33359,10.);
#9079=VECTOR('',#33362,10.);
#9080=VECTOR('',#33363,10.);
#9081=VECTOR('',#33366,10.);
#9082=VECTOR('',#33369,10.);
#9083=VECTOR('',#33374,2.5);
#9084=VECTOR('',#33381,2.5);
#9085=VECTOR('',#33388,2.5);
#9086=VECTOR('',#33393,10.);
#9087=VECTOR('',#33394,10.);
#9088=VECTOR('',#33395,10.);
#9089=VECTOR('',#33396,10.);
#9090=VECTOR('',#33399,10.);
#9091=VECTOR('',#33400,10.);
#9092=VECTOR('',#33401,10.);
#9093=VECTOR('',#33406,10.);
#9094=VECTOR('',#33411,10.);
#9095=VECTOR('',#33412,10.);
#9096=VECTOR('',#33413,10.);
#9097=VECTOR('',#33416,10.);
#9098=VECTOR('',#33423,10.);
#9099=VECTOR('',#33426,10.);
#9100=VECTOR('',#33429,10.);
#9101=VECTOR('',#33432,10.);
#9102=VECTOR('',#33435,10.);
#9103=VECTOR('',#33438,10.);
#9104=VECTOR('',#33441,10.);
#9105=VECTOR('',#33444,10.);
#9106=VECTOR('',#33447,10.);
#9107=VECTOR('',#33450,10.);
#9108=VECTOR('',#33455,10.);
#9109=VECTOR('',#33456,10.);
#9110=VECTOR('',#33457,10.);
#9111=VECTOR('',#33462,10.);
#9112=VECTOR('',#33467,10.);
#9113=VECTOR('',#33468,10.);
#9114=VECTOR('',#33469,10.);
#9115=VECTOR('',#33474,10.);
#9116=VECTOR('',#33479,10.);
#9117=VECTOR('',#33480,10.);
#9118=VECTOR('',#33481,10.);
#9119=VECTOR('',#33486,10.);
#9120=VECTOR('',#33491,10.);
#9121=VECTOR('',#33492,10.);
#9122=VECTOR('',#33493,10.);
#9123=VECTOR('',#33498,10.);
#9124=VECTOR('',#33503,10.);
#9125=VECTOR('',#33504,10.);
#9126=VECTOR('',#33505,10.);
#9127=VECTOR('',#33510,10.);
#9128=VECTOR('',#33515,10.);
#9129=VECTOR('',#33516,10.);
#9130=VECTOR('',#33517,10.);
#9131=VECTOR('',#33522,10.);
#9132=VECTOR('',#33527,10.);
#9133=VECTOR('',#33528,10.);
#9134=VECTOR('',#33529,10.);
#9135=VECTOR('',#33532,10.);
#9136=VECTOR('',#33533,10.);
#9137=VECTOR('',#33534,10.);
#9138=VECTOR('',#33537,10.);
#9139=VECTOR('',#33538,10.);
#9140=VECTOR('',#33539,10.);
#9141=VECTOR('',#33544,10.);
#9142=VECTOR('',#33549,10.);
#9143=VECTOR('',#33550,10.);
#9144=VECTOR('',#33551,10.);
#9145=VECTOR('',#33554,10.);
#9146=VECTOR('',#33555,10.);
#9147=VECTOR('',#33556,10.);
#9148=VECTOR('',#33559,10.);
#9149=VECTOR('',#33560,10.);
#9150=VECTOR('',#33563,10.);
#9151=VECTOR('',#33564,10.);
#9152=VECTOR('',#33565,10.);
#9153=VECTOR('',#33572,10.);
#9154=VECTOR('',#33575,10.);
#9155=VECTOR('',#33576,10.);
#9156=VECTOR('',#33577,10.);
#9157=VECTOR('',#33580,10.);
#9158=VECTOR('',#33587,10.);
#9159=VECTOR('',#33588,10.);
#9160=VECTOR('',#33591,10.);
#9161=VECTOR('',#33596,10.);
#9162=VECTOR('',#33597,10.);
#9163=VECTOR('',#33600,10.);
#9164=VECTOR('',#33605,10.);
#9165=VECTOR('',#33606,10.);
#9166=VECTOR('',#33609,10.);
#9167=VECTOR('',#33614,10.);
#9168=VECTOR('',#33615,10.);
#9169=VECTOR('',#33618,10.);
#9170=VECTOR('',#33623,10.);
#9171=VECTOR('',#33624,10.);
#9172=VECTOR('',#33627,10.);
#9173=VECTOR('',#33632,10.);
#9174=VECTOR('',#33635,10.);
#9175=VECTOR('',#33636,10.);
#9176=VECTOR('',#33637,10.);
#9177=VECTOR('',#33644,10.);
#9178=VECTOR('',#33647,10.);
#9179=VECTOR('',#33648,10.);
#9180=VECTOR('',#33649,10.);
#9181=VECTOR('',#33656,10.);
#9182=VECTOR('',#33659,10.);
#9183=VECTOR('',#33660,10.);
#9184=VECTOR('',#33661,10.);
#9185=VECTOR('',#33668,10.);
#9186=VECTOR('',#33671,10.);
#9187=VECTOR('',#33672,10.);
#9188=VECTOR('',#33673,10.);
#9189=VECTOR('',#33680,10.);
#9190=VECTOR('',#33683,10.);
#9191=VECTOR('',#33684,10.);
#9192=VECTOR('',#33685,10.);
#9193=VECTOR('',#33692,10.);
#9194=VECTOR('',#33695,10.);
#9195=VECTOR('',#33696,10.);
#9196=VECTOR('',#33697,10.);
#9197=VECTOR('',#33704,10.);
#9198=VECTOR('',#33707,10.);
#9199=VECTOR('',#33708,10.);
#9200=VECTOR('',#33709,10.);
#9201=VECTOR('',#33712,10.);
#9202=VECTOR('',#33713,10.);
#9203=VECTOR('',#33714,10.);
#9204=VECTOR('',#33717,10.);
#9205=VECTOR('',#33718,10.);
#9206=VECTOR('',#33719,10.);
#9207=VECTOR('',#33726,10.);
#9208=VECTOR('',#33729,10.);
#9209=VECTOR('',#33730,10.);
#9210=VECTOR('',#33731,10.);
#9211=VECTOR('',#33734,10.);
#9212=VECTOR('',#33735,10.);
#9213=VECTOR('',#33736,10.);
#9214=VECTOR('',#33739,10.);
#9215=VECTOR('',#33740,10.);
#11436=VERTEX_POINT('',#125619);
#11437=VERTEX_POINT('',#125620);
#11438=VERTEX_POINT('',#125623);
#11439=VERTEX_POINT('',#125628);
#11440=VERTEX_POINT('',#125629);
#11441=VERTEX_POINT('',#125632);
#11442=VERTEX_POINT('',#125638);
#11443=VERTEX_POINT('',#125640);
#11444=VERTEX_POINT('',#125642);
#11445=VERTEX_POINT('',#125644);
#11446=VERTEX_POINT('',#125648);
#11447=VERTEX_POINT('',#125649);
#11448=VERTEX_POINT('',#125653);
#11449=VERTEX_POINT('',#125655);
#11450=VERTEX_POINT('',#125657);
#11451=VERTEX_POINT('',#125662);
#11452=VERTEX_POINT('',#125664);
#11453=VERTEX_POINT('',#125675);
#11454=VERTEX_POINT('',#125677);
#11455=VERTEX_POINT('',#125704);
#11456=VERTEX_POINT('',#125706);
#11457=VERTEX_POINT('',#125717);
#11458=VERTEX_POINT('',#125719);
#11459=VERTEX_POINT('',#125726);
#11460=VERTEX_POINT('',#125728);
#11461=VERTEX_POINT('',#125735);
#11462=VERTEX_POINT('',#125737);
#11463=VERTEX_POINT('',#125744);
#11464=VERTEX_POINT('',#125746);
#11465=VERTEX_POINT('',#125763);
#11466=VERTEX_POINT('',#125765);
#11467=VERTEX_POINT('',#125792);
#11468=VERTEX_POINT('',#125794);
#11469=VERTEX_POINT('',#125811);
#11470=VERTEX_POINT('',#125813);
#11471=VERTEX_POINT('',#125815);
#11472=VERTEX_POINT('',#125817);
#11473=VERTEX_POINT('',#125834);
#11474=VERTEX_POINT('',#125836);
#11475=VERTEX_POINT('',#125863);
#11476=VERTEX_POINT('',#125865);
#11477=VERTEX_POINT('',#125882);
#11478=VERTEX_POINT('',#125884);
#11479=VERTEX_POINT('',#125893);
#11480=VERTEX_POINT('',#125895);
#11481=VERTEX_POINT('',#125902);
#11482=VERTEX_POINT('',#125904);
#11483=VERTEX_POINT('',#125915);
#11484=VERTEX_POINT('',#125917);
#11485=VERTEX_POINT('',#125932);
#11486=VERTEX_POINT('',#125934);
#11487=VERTEX_POINT('',#125966);
#11488=VERTEX_POINT('',#125968);
#11489=VERTEX_POINT('',#125983);
#11490=VERTEX_POINT('',#125985);
#11491=VERTEX_POINT('',#125992);
#11492=VERTEX_POINT('',#125996);
#11493=VERTEX_POINT('',#126005);
#11494=VERTEX_POINT('',#126007);
#11495=VERTEX_POINT('',#126014);
#11496=VERTEX_POINT('',#126016);
#11497=VERTEX_POINT('',#126027);
#11498=VERTEX_POINT('',#126029);
#11499=VERTEX_POINT('',#126036);
#11500=VERTEX_POINT('',#126038);
#11501=VERTEX_POINT('',#126045);
#11502=VERTEX_POINT('',#126054);
#11503=VERTEX_POINT('',#126055);
#11504=VERTEX_POINT('',#126059);
#11505=VERTEX_POINT('',#126061);
#11506=VERTEX_POINT('',#126063);
#11507=VERTEX_POINT('',#126068);
#11508=VERTEX_POINT('',#126070);
#11509=VERTEX_POINT('',#126081);
#11510=VERTEX_POINT('',#126083);
#11511=VERTEX_POINT('',#126110);
#11512=VERTEX_POINT('',#126112);
#11513=VERTEX_POINT('',#126123);
#11514=VERTEX_POINT('',#126125);
#11515=VERTEX_POINT('',#126132);
#11516=VERTEX_POINT('',#126134);
#11517=VERTEX_POINT('',#126141);
#11518=VERTEX_POINT('',#126143);
#11519=VERTEX_POINT('',#126150);
#11520=VERTEX_POINT('',#126152);
#11521=VERTEX_POINT('',#126169);
#11522=VERTEX_POINT('',#126171);
#11523=VERTEX_POINT('',#126198);
#11524=VERTEX_POINT('',#126200);
#11525=VERTEX_POINT('',#126217);
#11526=VERTEX_POINT('',#126219);
#11527=VERTEX_POINT('',#126221);
#11528=VERTEX_POINT('',#126223);
#11529=VERTEX_POINT('',#126240);
#11530=VERTEX_POINT('',#126242);
#11531=VERTEX_POINT('',#126269);
#11532=VERTEX_POINT('',#126271);
#11533=VERTEX_POINT('',#126288);
#11534=VERTEX_POINT('',#126290);
#11535=VERTEX_POINT('',#126299);
#11536=VERTEX_POINT('',#126301);
#11537=VERTEX_POINT('',#126308);
#11538=VERTEX_POINT('',#126310);
#11539=VERTEX_POINT('',#126321);
#11540=VERTEX_POINT('',#126323);
#11541=VERTEX_POINT('',#126338);
#11542=VERTEX_POINT('',#126340);
#11543=VERTEX_POINT('',#126372);
#11544=VERTEX_POINT('',#126374);
#11545=VERTEX_POINT('',#126389);
#11546=VERTEX_POINT('',#126391);
#11547=VERTEX_POINT('',#126398);
#11548=VERTEX_POINT('',#126402);
#11549=VERTEX_POINT('',#126411);
#11550=VERTEX_POINT('',#126413);
#11551=VERTEX_POINT('',#126420);
#11552=VERTEX_POINT('',#126422);
#11553=VERTEX_POINT('',#126433);
#11554=VERTEX_POINT('',#126435);
#11555=VERTEX_POINT('',#126442);
#11556=VERTEX_POINT('',#126444);
#11557=VERTEX_POINT('',#126451);
#11558=VERTEX_POINT('',#126460);
#11559=VERTEX_POINT('',#126461);
#11560=VERTEX_POINT('',#126465);
#11561=VERTEX_POINT('',#126467);
#11562=VERTEX_POINT('',#126469);
#11563=VERTEX_POINT('',#126474);
#11564=VERTEX_POINT('',#126476);
#11565=VERTEX_POINT('',#126489);
#11566=VERTEX_POINT('',#126491);
#11567=VERTEX_POINT('',#126518);
#11568=VERTEX_POINT('',#126520);
#11569=VERTEX_POINT('',#126533);
#11570=VERTEX_POINT('',#126535);
#11571=VERTEX_POINT('',#126542);
#11572=VERTEX_POINT('',#126544);
#11573=VERTEX_POINT('',#126551);
#11574=VERTEX_POINT('',#126553);
#11575=VERTEX_POINT('',#126560);
#11576=VERTEX_POINT('',#126562);
#11577=VERTEX_POINT('',#126579);
#11578=VERTEX_POINT('',#126581);
#11579=VERTEX_POINT('',#126608);
#11580=VERTEX_POINT('',#126610);
#11581=VERTEX_POINT('',#126627);
#11582=VERTEX_POINT('',#126629);
#11583=VERTEX_POINT('',#126631);
#11584=VERTEX_POINT('',#126633);
#11585=VERTEX_POINT('',#126650);
#11586=VERTEX_POINT('',#126652);
#11587=VERTEX_POINT('',#126679);
#11588=VERTEX_POINT('',#126681);
#11589=VERTEX_POINT('',#126698);
#11590=VERTEX_POINT('',#126700);
#11591=VERTEX_POINT('',#126709);
#11592=VERTEX_POINT('',#126711);
#11593=VERTEX_POINT('',#126718);
#11594=VERTEX_POINT('',#126720);
#11595=VERTEX_POINT('',#126731);
#11596=VERTEX_POINT('',#126733);
#11597=VERTEX_POINT('',#126748);
#11598=VERTEX_POINT('',#126750);
#11599=VERTEX_POINT('',#126782);
#11600=VERTEX_POINT('',#126784);
#11601=VERTEX_POINT('',#126799);
#11602=VERTEX_POINT('',#126801);
#11603=VERTEX_POINT('',#126808);
#11604=VERTEX_POINT('',#126812);
#11605=VERTEX_POINT('',#126821);
#11606=VERTEX_POINT('',#126823);
#11607=VERTEX_POINT('',#126830);
#11608=VERTEX_POINT('',#126832);
#11609=VERTEX_POINT('',#126843);
#11610=VERTEX_POINT('',#126845);
#11611=VERTEX_POINT('',#126852);
#11612=VERTEX_POINT('',#126854);
#11613=VERTEX_POINT('',#126861);
#11614=VERTEX_POINT('',#126870);
#11615=VERTEX_POINT('',#126872);
#11616=VERTEX_POINT('',#126874);
#11617=VERTEX_POINT('',#126876);
#11618=VERTEX_POINT('',#126882);
#11619=VERTEX_POINT('',#126886);
#11620=VERTEX_POINT('',#126892);
#11621=VERTEX_POINT('',#126896);
#11622=VERTEX_POINT('',#126902);
#11623=VERTEX_POINT('',#126906);
#11624=VERTEX_POINT('',#126912);
#11625=VERTEX_POINT('',#126916);
#11626=VERTEX_POINT('',#126922);
#11627=VERTEX_POINT('',#126926);
#11628=VERTEX_POINT('',#126932);
#11629=VERTEX_POINT('',#126936);
#11630=VERTEX_POINT('',#126942);
#11631=VERTEX_POINT('',#126946);
#11632=VERTEX_POINT('',#126952);
#11633=VERTEX_POINT('',#126956);
#11634=VERTEX_POINT('',#126962);
#11635=VERTEX_POINT('',#126966);
#11636=VERTEX_POINT('',#126972);
#11637=VERTEX_POINT('',#126976);
#11638=VERTEX_POINT('',#126982);
#11639=VERTEX_POINT('',#126986);
#11640=VERTEX_POINT('',#126994);
#11641=VERTEX_POINT('',#126996);
#11642=VERTEX_POINT('',#126998);
#11643=VERTEX_POINT('',#127000);
#11644=VERTEX_POINT('',#127004);
#11645=VERTEX_POINT('',#127012);
#11646=VERTEX_POINT('',#127020);
#11647=VERTEX_POINT('',#127028);
#11648=VERTEX_POINT('',#127036);
#11649=VERTEX_POINT('',#127044);
#11650=VERTEX_POINT('',#127052);
#11651=VERTEX_POINT('',#127060);
#11652=VERTEX_POINT('',#127068);
#11653=VERTEX_POINT('',#127076);
#11654=VERTEX_POINT('',#127084);
#11655=VERTEX_POINT('',#127092);
#11656=VERTEX_POINT('',#127094);
#11657=VERTEX_POINT('',#127098);
#11658=VERTEX_POINT('',#127100);
#11659=VERTEX_POINT('',#127104);
#11660=VERTEX_POINT('',#127106);
#11661=VERTEX_POINT('',#127110);
#11662=VERTEX_POINT('',#127111);
#11663=VERTEX_POINT('',#127113);
#11664=VERTEX_POINT('',#127115);
#11665=VERTEX_POINT('',#127119);
#11666=VERTEX_POINT('',#127121);
#11667=VERTEX_POINT('',#127125);
#11668=VERTEX_POINT('',#127127);
#11669=VERTEX_POINT('',#127131);
#11670=VERTEX_POINT('',#127133);
#11671=VERTEX_POINT('',#127162);
#11672=VERTEX_POINT('',#127164);
#11673=VERTEX_POINT('',#127168);
#11674=VERTEX_POINT('',#127170);
#11675=VERTEX_POINT('',#127174);
#11676=VERTEX_POINT('',#127176);
#11677=VERTEX_POINT('',#127180);
#11678=VERTEX_POINT('',#127182);
#11679=VERTEX_POINT('',#127186);
#11680=VERTEX_POINT('',#127188);
#11681=VERTEX_POINT('',#127192);
#11682=VERTEX_POINT('',#127194);
#11683=VERTEX_POINT('',#127198);
#11684=VERTEX_POINT('',#127200);
#11685=VERTEX_POINT('',#127204);
#11686=VERTEX_POINT('',#127206);
#11687=VERTEX_POINT('',#127210);
#11688=VERTEX_POINT('',#127212);
#11689=VERTEX_POINT('',#127216);
#11690=VERTEX_POINT('',#127218);
#11691=VERTEX_POINT('',#127222);
#11692=VERTEX_POINT('',#127224);
#11693=VERTEX_POINT('',#127228);
#11694=VERTEX_POINT('',#127230);
#11695=VERTEX_POINT('',#127234);
#11696=VERTEX_POINT('',#127236);
#11697=VERTEX_POINT('',#127240);
#11698=VERTEX_POINT('',#127242);
#11699=VERTEX_POINT('',#127246);
#11700=VERTEX_POINT('',#127248);
#11701=VERTEX_POINT('',#127252);
#11702=VERTEX_POINT('',#127254);
#11703=VERTEX_POINT('',#127258);
#11704=VERTEX_POINT('',#127260);
#11705=VERTEX_POINT('',#127264);
#11706=VERTEX_POINT('',#127266);
#11707=VERTEX_POINT('',#127273);
#11708=VERTEX_POINT('',#127275);
#11709=VERTEX_POINT('',#127279);
#11710=VERTEX_POINT('',#127281);
#11711=VERTEX_POINT('',#127285);
#11712=VERTEX_POINT('',#127287);
#11713=VERTEX_POINT('',#127291);
#11714=VERTEX_POINT('',#127296);
#11715=VERTEX_POINT('',#127300);
#11716=VERTEX_POINT('',#127304);
#11717=VERTEX_POINT('',#127308);
#11718=VERTEX_POINT('',#127312);
#11719=VERTEX_POINT('',#127316);
#11720=VERTEX_POINT('',#127320);
#11721=VERTEX_POINT('',#127324);
#11722=VERTEX_POINT('',#127328);
#11723=VERTEX_POINT('',#127332);
#11724=VERTEX_POINT('',#127338);
#11725=VERTEX_POINT('',#127340);
#11726=VERTEX_POINT('',#127344);
#11727=VERTEX_POINT('',#127346);
#11728=VERTEX_POINT('',#127350);
#11729=VERTEX_POINT('',#127352);
#11730=VERTEX_POINT('',#127356);
#11731=VERTEX_POINT('',#127358);
#11732=VERTEX_POINT('',#127362);
#11733=VERTEX_POINT('',#127364);
#11734=VERTEX_POINT('',#127368);
#11735=VERTEX_POINT('',#127370);
#11736=VERTEX_POINT('',#127374);
#11737=VERTEX_POINT('',#127376);
#11738=VERTEX_POINT('',#127380);
#11739=VERTEX_POINT('',#127382);
#11740=VERTEX_POINT('',#127386);
#11741=VERTEX_POINT('',#127388);
#11742=VERTEX_POINT('',#127392);
#11743=VERTEX_POINT('',#127394);
#11744=VERTEX_POINT('',#127398);
#11745=VERTEX_POINT('',#127400);
#11746=VERTEX_POINT('',#127404);
#11747=VERTEX_POINT('',#127406);
#11748=VERTEX_POINT('',#127410);
#11749=VERTEX_POINT('',#127412);
#11750=VERTEX_POINT('',#127416);
#11751=VERTEX_POINT('',#127418);
#11752=VERTEX_POINT('',#127422);
#11753=VERTEX_POINT('',#127424);
#11754=VERTEX_POINT('',#127428);
#11755=VERTEX_POINT('',#127430);
#11756=VERTEX_POINT('',#127434);
#11757=VERTEX_POINT('',#127436);
#11758=VERTEX_POINT('',#127440);
#11759=VERTEX_POINT('',#127442);
#15178=EDGE_CURVE('',#11436,#11437,#5992,.T.);
#15179=EDGE_CURVE('',#11437,#11436,#5993,.T.);
#15180=EDGE_CURVE('',#11437,#11438,#7088,.T.);
#15181=EDGE_CURVE('',#11438,#11438,#5994,.T.);
#15182=EDGE_CURVE('',#11439,#11440,#5995,.T.);
#15183=EDGE_CURVE('',#11440,#11439,#5996,.T.);
#15184=EDGE_CURVE('',#11440,#11441,#7089,.T.);
#15185=EDGE_CURVE('',#11441,#11441,#5997,.T.);
#15186=EDGE_CURVE('',#11437,#11439,#7090,.T.);
#15187=EDGE_CURVE('',#11440,#11442,#7091,.T.);
#15188=EDGE_CURVE('',#11443,#11442,#7092,.T.);
#15189=EDGE_CURVE('',#11444,#11443,#7093,.T.);
#15190=EDGE_CURVE('',#11444,#11445,#7094,.T.);
#15191=EDGE_CURVE('',#11445,#11436,#7095,.T.);
#15192=EDGE_CURVE('',#11446,#11447,#7096,.T.);
#15193=EDGE_CURVE('',#11447,#11446,#5998,.T.);
#15194=EDGE_CURVE('',#11448,#11448,#5999,.T.);
#15195=EDGE_CURVE('',#11448,#11449,#7097,.T.);
#15196=EDGE_CURVE('',#11450,#11449,#1155,.F.);
#15197=EDGE_CURVE('',#11451,#11450,#6000,.T.);
#15198=EDGE_CURVE('',#11452,#11451,#1156,.T.);
#15199=EDGE_CURVE('',#11453,#11452,#7098,.T.);
#15200=EDGE_CURVE('',#11454,#11453,#1157,.T.);
#15201=EDGE_CURVE('',#11455,#11454,#7099,.T.);
#15202=EDGE_CURVE('',#11456,#11455,#1158,.T.);
#15203=EDGE_CURVE('',#11457,#11456,#6001,.T.);
#15204=EDGE_CURVE('',#11458,#11457,#1159,.T.);
#15205=EDGE_CURVE('',#11459,#11458,#119,.T.);
#15206=EDGE_CURVE('',#11460,#11459,#1160,.T.);
#15207=EDGE_CURVE('',#11461,#11460,#7100,.T.);
#15208=EDGE_CURVE('',#11462,#11461,#1161,.T.);
#15209=EDGE_CURVE('',#11463,#11462,#120,.T.);
#15210=EDGE_CURVE('',#11464,#11463,#1162,.T.);
#15211=EDGE_CURVE('',#11465,#11464,#7101,.T.);
#15212=EDGE_CURVE('',#11466,#11465,#1163,.T.);
#15213=EDGE_CURVE('',#11467,#11466,#7102,.T.);
#15214=EDGE_CURVE('',#11468,#11467,#1164,.T.);
#15215=EDGE_CURVE('',#11469,#11468,#121,.T.);
#15216=EDGE_CURVE('',#11469,#11470,#7103,.T.);
#15217=EDGE_CURVE('',#11471,#11470,#122,.T.);
#15218=EDGE_CURVE('',#11472,#11471,#1165,.T.);
#15219=EDGE_CURVE('',#11473,#11472,#7104,.T.);
#15220=EDGE_CURVE('',#11474,#11473,#1166,.T.);
#15221=EDGE_CURVE('',#11475,#11474,#7105,.T.);
#15222=EDGE_CURVE('',#11476,#11475,#1167,.T.);
#15223=EDGE_CURVE('',#11477,#11476,#123,.T.);
#15224=EDGE_CURVE('',#11478,#11477,#1168,.T.);
#15225=EDGE_CURVE('',#11479,#11478,#7106,.T.);
#15226=EDGE_CURVE('',#11480,#11479,#1169,.T.);
#15227=EDGE_CURVE('',#11481,#11480,#124,.T.);
#15228=EDGE_CURVE('',#11482,#11481,#1170,.T.);
#15229=EDGE_CURVE('',#11483,#11482,#6002,.T.);
#15230=EDGE_CURVE('',#11484,#11483,#1171,.T.);
#15231=EDGE_CURVE('',#11485,#11484,#7107,.T.);
#15232=EDGE_CURVE('',#11486,#11485,#1172,.T.);
#15233=EDGE_CURVE('',#11487,#11486,#7108,.T.);
#15234=EDGE_CURVE('',#11488,#11487,#1173,.T.);
#15235=EDGE_CURVE('',#11489,#11488,#6003,.T.);
#15236=EDGE_CURVE('',#11490,#11489,#1174,.T.);
#15237=EDGE_CURVE('',#11490,#11491,#7109,.T.);
#15238=EDGE_CURVE('',#11447,#11491,#6004,.T.);
#15239=EDGE_CURVE('',#11491,#11446,#6005,.T.);
#15240=EDGE_CURVE('',#11492,#11490,#1175,.T.);
#15241=EDGE_CURVE('',#11493,#11492,#125,.T.);
#15242=EDGE_CURVE('',#11494,#11493,#1176,.T.);
#15243=EDGE_CURVE('',#11495,#11494,#7110,.T.);
#15244=EDGE_CURVE('',#11496,#11495,#1177,.T.);
#15245=EDGE_CURVE('',#11470,#11496,#126,.T.);
#15246=EDGE_CURVE('',#11497,#11469,#127,.T.);
#15247=EDGE_CURVE('',#11498,#11497,#1178,.T.);
#15248=EDGE_CURVE('',#11499,#11498,#7111,.T.);
#15249=EDGE_CURVE('',#11500,#11499,#1179,.T.);
#15250=EDGE_CURVE('',#11501,#11500,#128,.T.);
#15251=EDGE_CURVE('',#11449,#11501,#1180,.F.);
#15252=EDGE_CURVE('',#11502,#11503,#7112,.T.);
#15253=EDGE_CURVE('',#11503,#11502,#6006,.T.);
#15254=EDGE_CURVE('',#11504,#11504,#6007,.T.);
#15255=EDGE_CURVE('',#11504,#11505,#7113,.T.);
#15256=EDGE_CURVE('',#11506,#11505,#1181,.F.);
#15257=EDGE_CURVE('',#11507,#11506,#6008,.T.);
#15258=EDGE_CURVE('',#11508,#11507,#1182,.T.);
#15259=EDGE_CURVE('',#11509,#11508,#7114,.T.);
#15260=EDGE_CURVE('',#11510,#11509,#1183,.T.);
#15261=EDGE_CURVE('',#11511,#11510,#7115,.T.);
#15262=EDGE_CURVE('',#11512,#11511,#1184,.T.);
#15263=EDGE_CURVE('',#11513,#11512,#6009,.T.);
#15264=EDGE_CURVE('',#11514,#11513,#1185,.T.);
#15265=EDGE_CURVE('',#11515,#11514,#129,.T.);
#15266=EDGE_CURVE('',#11516,#11515,#1186,.T.);
#15267=EDGE_CURVE('',#11517,#11516,#7116,.T.);
#15268=EDGE_CURVE('',#11518,#11517,#1187,.T.);
#15269=EDGE_CURVE('',#11519,#11518,#130,.T.);
#15270=EDGE_CURVE('',#11520,#11519,#1188,.T.);
#15271=EDGE_CURVE('',#11521,#11520,#7117,.T.);
#15272=EDGE_CURVE('',#11522,#11521,#1189,.T.);
#15273=EDGE_CURVE('',#11523,#11522,#7118,.T.);
#15274=EDGE_CURVE('',#11524,#11523,#1190,.T.);
#15275=EDGE_CURVE('',#11525,#11524,#131,.T.);
#15276=EDGE_CURVE('',#11525,#11526,#7119,.T.);
#15277=EDGE_CURVE('',#11527,#11526,#132,.T.);
#15278=EDGE_CURVE('',#11528,#11527,#1191,.T.);
#15279=EDGE_CURVE('',#11529,#11528,#7120,.T.);
#15280=EDGE_CURVE('',#11530,#11529,#1192,.T.);
#15281=EDGE_CURVE('',#11531,#11530,#7121,.T.);
#15282=EDGE_CURVE('',#11532,#11531,#1193,.T.);
#15283=EDGE_CURVE('',#11533,#11532,#133,.T.);
#15284=EDGE_CURVE('',#11534,#11533,#1194,.T.);
#15285=EDGE_CURVE('',#11535,#11534,#7122,.T.);
#15286=EDGE_CURVE('',#11536,#11535,#1195,.T.);
#15287=EDGE_CURVE('',#11537,#11536,#134,.T.);
#15288=EDGE_CURVE('',#11538,#11537,#1196,.T.);
#15289=EDGE_CURVE('',#11539,#11538,#6010,.T.);
#15290=EDGE_CURVE('',#11540,#11539,#1197,.T.);
#15291=EDGE_CURVE('',#11541,#11540,#7123,.T.);
#15292=EDGE_CURVE('',#11542,#11541,#1198,.T.);
#15293=EDGE_CURVE('',#11543,#11542,#7124,.T.);
#15294=EDGE_CURVE('',#11544,#11543,#1199,.T.);
#15295=EDGE_CURVE('',#11545,#11544,#6011,.T.);
#15296=EDGE_CURVE('',#11546,#11545,#1200,.T.);
#15297=EDGE_CURVE('',#11546,#11547,#7125,.T.);
#15298=EDGE_CURVE('',#11503,#11547,#6012,.T.);
#15299=EDGE_CURVE('',#11547,#11502,#6013,.T.);
#15300=EDGE_CURVE('',#11548,#11546,#1201,.T.);
#15301=EDGE_CURVE('',#11549,#11548,#135,.T.);
#15302=EDGE_CURVE('',#11550,#11549,#1202,.T.);
#15303=EDGE_CURVE('',#11551,#11550,#7126,.T.);
#15304=EDGE_CURVE('',#11552,#11551,#1203,.T.);
#15305=EDGE_CURVE('',#11526,#11552,#136,.T.);
#15306=EDGE_CURVE('',#11553,#11525,#137,.T.);
#15307=EDGE_CURVE('',#11554,#11553,#1204,.T.);
#15308=EDGE_CURVE('',#11555,#11554,#7127,.T.);
#15309=EDGE_CURVE('',#11556,#11555,#1205,.T.);
#15310=EDGE_CURVE('',#11557,#11556,#138,.T.);
#15311=EDGE_CURVE('',#11505,#11557,#1206,.F.);
#15312=EDGE_CURVE('',#11558,#11559,#7128,.T.);
#15313=EDGE_CURVE('',#11559,#11558,#6014,.T.);
#15314=EDGE_CURVE('',#11560,#11560,#6015,.T.);
#15315=EDGE_CURVE('',#11560,#11561,#7129,.T.);
#15316=EDGE_CURVE('',#11562,#11561,#1207,.F.);
#15317=EDGE_CURVE('',#11563,#11562,#6016,.T.);
#15318=EDGE_CURVE('',#11564,#11563,#1208,.T.);
#15319=EDGE_CURVE('',#11565,#11564,#7130,.T.);
#15320=EDGE_CURVE('',#11566,#11565,#1209,.T.);
#15321=EDGE_CURVE('',#11567,#11566,#7131,.T.);
#15322=EDGE_CURVE('',#11568,#11567,#1210,.T.);
#15323=EDGE_CURVE('',#11569,#11568,#6017,.T.);
#15324=EDGE_CURVE('',#11570,#11569,#1211,.T.);
#15325=EDGE_CURVE('',#11571,#11570,#139,.T.);
#15326=EDGE_CURVE('',#11572,#11571,#1212,.T.);
#15327=EDGE_CURVE('',#11573,#11572,#7132,.T.);
#15328=EDGE_CURVE('',#11574,#11573,#1213,.T.);
#15329=EDGE_CURVE('',#11575,#11574,#140,.T.);
#15330=EDGE_CURVE('',#11576,#11575,#1214,.T.);
#15331=EDGE_CURVE('',#11577,#11576,#7133,.T.);
#15332=EDGE_CURVE('',#11578,#11577,#1215,.T.);
#15333=EDGE_CURVE('',#11579,#11578,#7134,.T.);
#15334=EDGE_CURVE('',#11580,#11579,#1216,.T.);
#15335=EDGE_CURVE('',#11581,#11580,#141,.T.);
#15336=EDGE_CURVE('',#11581,#11582,#7135,.T.);
#15337=EDGE_CURVE('',#11583,#11582,#142,.T.);
#15338=EDGE_CURVE('',#11584,#11583,#1217,.T.);
#15339=EDGE_CURVE('',#11585,#11584,#7136,.T.);
#15340=EDGE_CURVE('',#11586,#11585,#1218,.T.);
#15341=EDGE_CURVE('',#11587,#11586,#7137,.T.);
#15342=EDGE_CURVE('',#11588,#11587,#1219,.T.);
#15343=EDGE_CURVE('',#11589,#11588,#143,.T.);
#15344=EDGE_CURVE('',#11590,#11589,#1220,.T.);
#15345=EDGE_CURVE('',#11591,#11590,#7138,.T.);
#15346=EDGE_CURVE('',#11592,#11591,#1221,.T.);
#15347=EDGE_CURVE('',#11593,#11592,#144,.T.);
#15348=EDGE_CURVE('',#11594,#11593,#1222,.T.);
#15349=EDGE_CURVE('',#11595,#11594,#6018,.T.);
#15350=EDGE_CURVE('',#11596,#11595,#1223,.T.);
#15351=EDGE_CURVE('',#11597,#11596,#7139,.T.);
#15352=EDGE_CURVE('',#11598,#11597,#1224,.T.);
#15353=EDGE_CURVE('',#11599,#11598,#7140,.T.);
#15354=EDGE_CURVE('',#11600,#11599,#1225,.T.);
#15355=EDGE_CURVE('',#11601,#11600,#6019,.T.);
#15356=EDGE_CURVE('',#11602,#11601,#1226,.T.);
#15357=EDGE_CURVE('',#11602,#11603,#7141,.T.);
#15358=EDGE_CURVE('',#11559,#11603,#6020,.T.);
#15359=EDGE_CURVE('',#11603,#11558,#6021,.T.);
#15360=EDGE_CURVE('',#11604,#11602,#1227,.T.);
#15361=EDGE_CURVE('',#11605,#11604,#145,.T.);
#15362=EDGE_CURVE('',#11606,#11605,#1228,.T.);
#15363=EDGE_CURVE('',#11607,#11606,#7142,.T.);
#15364=EDGE_CURVE('',#11608,#11607,#1229,.T.);
#15365=EDGE_CURVE('',#11582,#11608,#146,.T.);
#15366=EDGE_CURVE('',#11609,#11581,#147,.T.);
#15367=EDGE_CURVE('',#11610,#11609,#1230,.T.);
#15368=EDGE_CURVE('',#11611,#11610,#7143,.T.);
#15369=EDGE_CURVE('',#11612,#11611,#1231,.T.);
#15370=EDGE_CURVE('',#11613,#11612,#148,.T.);
#15371=EDGE_CURVE('',#11561,#11613,#1232,.F.);
#15372=EDGE_CURVE('',#11614,#11453,#7144,.T.);
#15373=EDGE_CURVE('',#11615,#11614,#6022,.T.);
#15374=EDGE_CURVE('',#11615,#11616,#7145,.T.);
#15375=EDGE_CURVE('',#11616,#11617,#6023,.T.);
#15376=EDGE_CURVE('',#11566,#11617,#7146,.T.);
#15377=EDGE_CURVE('',#11510,#11565,#7147,.T.);
#15378=EDGE_CURVE('',#11454,#11509,#7148,.T.);
#15379=EDGE_CURVE('',#11618,#11452,#7149,.T.);
#15380=EDGE_CURVE('',#11614,#11618,#7150,.T.);
#15381=EDGE_CURVE('',#11617,#11619,#7151,.T.);
#15382=EDGE_CURVE('',#11567,#11619,#7152,.T.);
#15383=EDGE_CURVE('',#11511,#11564,#7153,.T.);
#15384=EDGE_CURVE('',#11620,#11451,#7154,.T.);
#15385=EDGE_CURVE('',#11620,#11618,#6024,.T.);
#15386=EDGE_CURVE('',#11619,#11621,#6025,.T.);
#15387=EDGE_CURVE('',#11568,#11621,#7155,.T.);
#15388=EDGE_CURVE('',#11512,#11563,#7156,.T.);
#15389=EDGE_CURVE('',#11622,#11450,#7157,.T.);
#15390=EDGE_CURVE('',#11620,#11622,#7158,.T.);
#15391=EDGE_CURVE('',#11621,#11623,#7159,.T.);
#15392=EDGE_CURVE('',#11569,#11623,#7160,.T.);
#15393=EDGE_CURVE('',#11513,#11562,#7161,.T.);
#15394=EDGE_CURVE('',#11624,#11501,#7162,.T.);
#15395=EDGE_CURVE('',#11624,#11622,#6026,.T.);
#15396=EDGE_CURVE('',#11623,#11625,#6027,.T.);
#15397=EDGE_CURVE('',#11570,#11625,#7163,.T.);
#15398=EDGE_CURVE('',#11514,#11613,#7164,.T.);
#15399=EDGE_CURVE('',#11626,#11500,#7165,.T.);
#15400=EDGE_CURVE('',#11624,#11626,#7166,.T.);
#15401=EDGE_CURVE('',#11625,#11627,#7167,.T.);
#15402=EDGE_CURVE('',#11571,#11627,#7168,.T.);
#15403=EDGE_CURVE('',#11515,#11612,#7169,.T.);
#15404=EDGE_CURVE('',#11628,#11499,#7170,.T.);
#15405=EDGE_CURVE('',#11628,#11626,#6028,.T.);
#15406=EDGE_CURVE('',#11627,#11629,#6029,.T.);
#15407=EDGE_CURVE('',#11572,#11629,#7171,.T.);
#15408=EDGE_CURVE('',#11516,#11611,#7172,.T.);
#15409=EDGE_CURVE('',#11630,#11498,#7173,.T.);
#15410=EDGE_CURVE('',#11628,#11630,#7174,.T.);
#15411=EDGE_CURVE('',#11629,#11631,#7175,.T.);
#15412=EDGE_CURVE('',#11573,#11631,#7176,.T.);
#15413=EDGE_CURVE('',#11517,#11610,#7177,.T.);
#15414=EDGE_CURVE('',#11632,#11497,#7178,.T.);
#15415=EDGE_CURVE('',#11632,#11630,#6030,.T.);
#15416=EDGE_CURVE('',#11631,#11633,#6031,.T.);
#15417=EDGE_CURVE('',#11574,#11633,#7179,.T.);
#15418=EDGE_CURVE('',#11518,#11609,#7180,.T.);
#15419=EDGE_CURVE('',#11634,#11468,#7181,.T.);
#15420=EDGE_CURVE('',#11632,#11634,#7182,.T.);
#15421=EDGE_CURVE('',#11633,#11635,#7183,.T.);
#15422=EDGE_CURVE('',#11575,#11635,#7184,.T.);
#15423=EDGE_CURVE('',#11519,#11580,#7185,.T.);
#15424=EDGE_CURVE('',#11636,#11467,#7186,.T.);
#15425=EDGE_CURVE('',#11636,#11634,#6032,.T.);
#15426=EDGE_CURVE('',#11635,#11637,#6033,.T.);
#15427=EDGE_CURVE('',#11576,#11637,#7187,.T.);
#15428=EDGE_CURVE('',#11520,#11579,#7188,.T.);
#15429=EDGE_CURVE('',#11638,#11466,#7189,.T.);
#15430=EDGE_CURVE('',#11636,#11638,#7190,.T.);
#15431=EDGE_CURVE('',#11637,#11639,#7191,.T.);
#15432=EDGE_CURVE('',#11577,#11639,#7192,.T.);
#15433=EDGE_CURVE('',#11521,#11578,#7193,.T.);
#15434=EDGE_CURVE('',#11485,#11542,#7194,.T.);
#15435=EDGE_CURVE('',#11541,#11598,#7195,.T.);
#15436=EDGE_CURVE('',#11597,#11640,#7196,.T.);
#15437=EDGE_CURVE('',#11641,#11640,#6034,.T.);
#15438=EDGE_CURVE('',#11642,#11641,#7197,.T.);
#15439=EDGE_CURVE('',#11642,#11643,#6035,.T.);
#15440=EDGE_CURVE('',#11643,#11486,#7198,.T.);
#15441=EDGE_CURVE('',#11596,#11644,#7199,.T.);
#15442=EDGE_CURVE('',#11640,#11644,#7200,.T.);
#15443=EDGE_CURVE('',#11540,#11599,#7201,.T.);
#15444=EDGE_CURVE('',#11484,#11543,#7202,.T.);
#15445=EDGE_CURVE('',#11595,#11645,#7203,.T.);
#15446=EDGE_CURVE('',#11644,#11645,#6036,.T.);
#15447=EDGE_CURVE('',#11539,#11600,#7204,.T.);
#15448=EDGE_CURVE('',#11483,#11544,#7205,.T.);
#15449=EDGE_CURVE('',#11594,#11646,#7206,.T.);
#15450=EDGE_CURVE('',#11645,#11646,#7207,.T.);
#15451=EDGE_CURVE('',#11538,#11601,#7208,.T.);
#15452=EDGE_CURVE('',#11482,#11545,#7209,.T.);
#15453=EDGE_CURVE('',#11593,#11647,#7210,.T.);
#15454=EDGE_CURVE('',#11646,#11647,#6037,.T.);
#15455=EDGE_CURVE('',#11537,#11604,#7211,.T.);
#15456=EDGE_CURVE('',#11481,#11548,#7212,.T.);
#15457=EDGE_CURVE('',#11592,#11648,#7213,.T.);
#15458=EDGE_CURVE('',#11647,#11648,#7214,.T.);
#15459=EDGE_CURVE('',#11536,#11605,#7215,.T.);
#15460=EDGE_CURVE('',#11480,#11549,#7216,.T.);
#15461=EDGE_CURVE('',#11591,#11649,#7217,.T.);
#15462=EDGE_CURVE('',#11648,#11649,#6038,.T.);
#15463=EDGE_CURVE('',#11535,#11606,#7218,.T.);
#15464=EDGE_CURVE('',#11479,#11550,#7219,.T.);
#15465=EDGE_CURVE('',#11590,#11650,#7220,.T.);
#15466=EDGE_CURVE('',#11649,#11650,#7221,.T.);
#15467=EDGE_CURVE('',#11534,#11607,#7222,.T.);
#15468=EDGE_CURVE('',#11478,#11551,#7223,.T.);
#15469=EDGE_CURVE('',#11589,#11651,#7224,.T.);
#15470=EDGE_CURVE('',#11650,#11651,#6039,.T.);
#15471=EDGE_CURVE('',#11533,#11608,#7225,.T.);
#15472=EDGE_CURVE('',#11477,#11552,#7226,.T.);
#15473=EDGE_CURVE('',#11588,#11652,#7227,.T.);
#15474=EDGE_CURVE('',#11651,#11652,#7228,.T.);
#15475=EDGE_CURVE('',#11532,#11583,#7229,.T.);
#15476=EDGE_CURVE('',#11476,#11527,#7230,.T.);
#15477=EDGE_CURVE('',#11587,#11653,#7231,.T.);
#15478=EDGE_CURVE('',#11652,#11653,#6040,.T.);
#15479=EDGE_CURVE('',#11531,#11584,#7232,.T.);
#15480=EDGE_CURVE('',#11475,#11528,#7233,.T.);
#15481=EDGE_CURVE('',#11586,#11654,#7234,.T.);
#15482=EDGE_CURVE('',#11653,#11654,#7235,.T.);
#15483=EDGE_CURVE('',#11530,#11585,#7236,.T.);
#15484=EDGE_CURVE('',#11474,#11529,#7237,.T.);
#15485=EDGE_CURVE('',#11655,#11655,#6041,.T.);
#15486=EDGE_CURVE('',#11655,#11656,#7238,.T.);
#15487=EDGE_CURVE('',#11656,#11656,#6042,.T.);
#15488=EDGE_CURVE('',#11657,#11657,#6043,.T.);
#15489=EDGE_CURVE('',#11657,#11658,#7239,.T.);
#15490=EDGE_CURVE('',#11658,#11658,#6044,.T.);
#15491=EDGE_CURVE('',#11659,#11659,#6045,.T.);
#15492=EDGE_CURVE('',#11659,#11660,#7240,.T.);
#15493=EDGE_CURVE('',#11660,#11660,#6046,.T.);
#15494=EDGE_CURVE('',#11661,#11662,#7241,.T.);
#15495=EDGE_CURVE('',#11662,#11663,#7242,.T.);
#15496=EDGE_CURVE('',#11663,#11664,#7243,.T.);
#15497=EDGE_CURVE('',#11661,#11664,#7244,.T.);
#15498=EDGE_CURVE('',#11665,#11445,#7245,.T.);
#15499=EDGE_CURVE('',#11665,#11666,#7246,.T.);
#15500=EDGE_CURVE('',#11666,#11442,#7247,.T.);
#15501=EDGE_CURVE('',#11667,#11665,#6047,.T.);
#15502=EDGE_CURVE('',#11667,#11668,#7248,.T.);
#15503=EDGE_CURVE('',#11668,#11666,#6048,.T.);
#15504=EDGE_CURVE('',#11669,#11667,#7249,.T.);
#15505=EDGE_CURVE('',#11669,#11670,#7250,.T.);
#15506=EDGE_CURVE('',#11670,#11668,#7251,.T.);
#15507=EDGE_CURVE('',#11465,#11522,#7252,.T.);
#15508=EDGE_CURVE('',#11639,#11670,#6049,.T.);
#15509=EDGE_CURVE('',#11638,#11669,#6050,.T.);
#15510=EDGE_CURVE('',#11464,#11523,#7253,.T.);
#15511=EDGE_CURVE('',#11463,#11524,#7254,.T.);
#15512=EDGE_CURVE('',#11462,#11553,#7255,.T.);
#15513=EDGE_CURVE('',#11461,#11554,#7256,.T.);
#15514=EDGE_CURVE('',#11460,#11555,#7257,.T.);
#15515=EDGE_CURVE('',#11459,#11556,#7258,.T.);
#15516=EDGE_CURVE('',#11458,#11557,#7259,.T.);
#15517=EDGE_CURVE('',#11457,#11506,#7260,.T.);
#15518=EDGE_CURVE('',#11456,#11507,#7261,.T.);
#15519=EDGE_CURVE('',#11455,#11508,#7262,.T.);
#15520=EDGE_CURVE('',#11671,#11615,#7263,.T.);
#15521=EDGE_CURVE('',#11671,#11672,#7264,.T.);
#15522=EDGE_CURVE('',#11672,#11616,#7265,.T.);
#15523=EDGE_CURVE('',#11673,#11671,#6051,.T.);
#15524=EDGE_CURVE('',#11673,#11674,#7266,.T.);
#15525=EDGE_CURVE('',#11674,#11672,#6052,.T.);
#15526=EDGE_CURVE('',#11675,#11673,#7267,.T.);
#15527=EDGE_CURVE('',#11675,#11676,#7268,.T.);
#15528=EDGE_CURVE('',#11676,#11674,#7269,.T.);
#15529=EDGE_CURVE('',#11677,#11675,#6053,.T.);
#15530=EDGE_CURVE('',#11677,#11678,#7270,.T.);
#15531=EDGE_CURVE('',#11678,#11676,#6054,.T.);
#15532=EDGE_CURVE('',#11679,#11677,#7271,.T.);
#15533=EDGE_CURVE('',#11679,#11680,#7272,.T.);
#15534=EDGE_CURVE('',#11680,#11678,#7273,.T.);
#15535=EDGE_CURVE('',#11679,#11681,#6055,.T.);
#15536=EDGE_CURVE('',#11681,#11682,#7274,.T.);
#15537=EDGE_CURVE('',#11682,#11680,#6056,.T.);
#15538=EDGE_CURVE('',#11683,#11681,#7275,.T.);
#15539=EDGE_CURVE('',#11683,#11684,#7276,.T.);
#15540=EDGE_CURVE('',#11684,#11682,#7277,.T.);
#15541=EDGE_CURVE('',#11685,#11683,#6057,.T.);
#15542=EDGE_CURVE('',#11685,#11686,#7278,.T.);
#15543=EDGE_CURVE('',#11686,#11684,#6058,.T.);
#15544=EDGE_CURVE('',#11687,#11685,#7279,.T.);
#15545=EDGE_CURVE('',#11687,#11688,#7280,.T.);
#15546=EDGE_CURVE('',#11688,#11686,#7281,.T.);
#15547=EDGE_CURVE('',#11689,#11687,#6059,.T.);
#15548=EDGE_CURVE('',#11689,#11690,#7282,.T.);
#15549=EDGE_CURVE('',#11690,#11688,#6060,.T.);
#15550=EDGE_CURVE('',#11691,#11689,#7283,.T.);
#15551=EDGE_CURVE('',#11691,#11692,#7284,.T.);
#15552=EDGE_CURVE('',#11692,#11690,#7285,.T.);
#15553=EDGE_CURVE('',#11693,#11691,#6061,.T.);
#15554=EDGE_CURVE('',#11693,#11694,#7286,.T.);
#15555=EDGE_CURVE('',#11694,#11692,#6062,.T.);
#15556=EDGE_CURVE('',#11695,#11693,#7287,.T.);
#15557=EDGE_CURVE('',#11695,#11696,#7288,.T.);
#15558=EDGE_CURVE('',#11696,#11694,#7289,.T.);
#15559=EDGE_CURVE('',#11697,#11695,#7290,.T.);
#15560=EDGE_CURVE('',#11697,#11698,#7291,.T.);
#15561=EDGE_CURVE('',#11698,#11696,#7292,.T.);
#15562=EDGE_CURVE('',#11699,#11697,#7293,.T.);
#15563=EDGE_CURVE('',#11699,#11700,#7294,.T.);
#15564=EDGE_CURVE('',#11700,#11698,#7295,.T.);
#15565=EDGE_CURVE('',#11699,#11701,#6063,.T.);
#15566=EDGE_CURVE('',#11701,#11702,#7296,.T.);
#15567=EDGE_CURVE('',#11702,#11700,#6064,.T.);
#15568=EDGE_CURVE('',#11703,#11701,#7297,.T.);
#15569=EDGE_CURVE('',#11703,#11704,#7298,.T.);
#15570=EDGE_CURVE('',#11704,#11702,#7299,.T.);
#15571=EDGE_CURVE('',#11705,#11703,#7300,.T.);
#15572=EDGE_CURVE('',#11705,#11706,#7301,.T.);
#15573=EDGE_CURVE('',#11706,#11704,#7302,.T.);
#15574=EDGE_CURVE('',#11661,#11705,#7303,.T.);
#15575=EDGE_CURVE('',#11664,#11706,#7304,.T.);
#15576=EDGE_CURVE('',#11707,#11662,#7305,.T.);
#15577=EDGE_CURVE('',#11707,#11708,#7306,.T.);
#15578=EDGE_CURVE('',#11663,#11708,#7307,.T.);
#15579=EDGE_CURVE('',#11709,#11444,#6065,.T.);
#15580=EDGE_CURVE('',#11710,#11443,#6066,.T.);
#15581=EDGE_CURVE('',#11709,#11710,#7308,.T.);
#15582=EDGE_CURVE('',#11711,#11709,#7309,.T.);
#15583=EDGE_CURVE('',#11712,#11710,#7310,.T.);
#15584=EDGE_CURVE('',#11711,#11712,#7311,.T.);
#15585=EDGE_CURVE('',#11713,#11473,#7312,.T.);
#15586=EDGE_CURVE('',#11713,#11711,#6067,.T.);
#15587=EDGE_CURVE('',#11654,#11712,#6068,.T.);
#15588=EDGE_CURVE('',#11714,#11472,#7313,.T.);
#15589=EDGE_CURVE('',#11714,#11713,#7314,.T.);
#15590=EDGE_CURVE('',#11715,#11471,#7315,.T.);
#15591=EDGE_CURVE('',#11714,#11715,#6069,.T.);
#15592=EDGE_CURVE('',#11716,#11496,#7316,.T.);
#15593=EDGE_CURVE('',#11716,#11715,#7317,.T.);
#15594=EDGE_CURVE('',#11717,#11495,#7318,.T.);
#15595=EDGE_CURVE('',#11716,#11717,#6070,.T.);
#15596=EDGE_CURVE('',#11718,#11494,#7319,.T.);
#15597=EDGE_CURVE('',#11718,#11717,#7320,.T.);
#15598=EDGE_CURVE('',#11719,#11493,#7321,.T.);
#15599=EDGE_CURVE('',#11718,#11719,#6071,.T.);
#15600=EDGE_CURVE('',#11720,#11492,#7322,.T.);
#15601=EDGE_CURVE('',#11720,#11719,#7323,.T.);
#15602=EDGE_CURVE('',#11721,#11489,#7324,.T.);
#15603=EDGE_CURVE('',#11720,#11721,#6072,.T.);
#15604=EDGE_CURVE('',#11722,#11488,#7325,.T.);
#15605=EDGE_CURVE('',#11722,#11721,#7326,.T.);
#15606=EDGE_CURVE('',#11723,#11487,#7327,.T.);
#15607=EDGE_CURVE('',#11722,#11723,#6073,.T.);
#15608=EDGE_CURVE('',#11643,#11723,#7328,.T.);
#15609=EDGE_CURVE('',#11724,#11642,#7329,.T.);
#15610=EDGE_CURVE('',#11725,#11641,#7330,.T.);
#15611=EDGE_CURVE('',#11724,#11725,#7331,.T.);
#15612=EDGE_CURVE('',#11726,#11724,#6074,.T.);
#15613=EDGE_CURVE('',#11727,#11725,#6075,.T.);
#15614=EDGE_CURVE('',#11726,#11727,#7332,.T.);
#15615=EDGE_CURVE('',#11728,#11726,#7333,.T.);
#15616=EDGE_CURVE('',#11729,#11727,#7334,.T.);
#15617=EDGE_CURVE('',#11728,#11729,#7335,.T.);
#15618=EDGE_CURVE('',#11730,#11728,#6076,.T.);
#15619=EDGE_CURVE('',#11731,#11729,#6077,.T.);
#15620=EDGE_CURVE('',#11730,#11731,#7336,.T.);
#15621=EDGE_CURVE('',#11732,#11730,#7337,.T.);
#15622=EDGE_CURVE('',#11733,#11731,#7338,.T.);
#15623=EDGE_CURVE('',#11732,#11733,#7339,.T.);
#15624=EDGE_CURVE('',#11732,#11734,#6078,.T.);
#15625=EDGE_CURVE('',#11735,#11733,#6079,.T.);
#15626=EDGE_CURVE('',#11734,#11735,#7340,.T.);
#15627=EDGE_CURVE('',#11736,#11734,#7341,.T.);
#15628=EDGE_CURVE('',#11737,#11735,#7342,.T.);
#15629=EDGE_CURVE('',#11736,#11737,#7343,.T.);
#15630=EDGE_CURVE('',#11738,#11736,#6080,.T.);
#15631=EDGE_CURVE('',#11739,#11737,#6081,.T.);
#15632=EDGE_CURVE('',#11738,#11739,#7344,.T.);
#15633=EDGE_CURVE('',#11740,#11738,#7345,.T.);
#15634=EDGE_CURVE('',#11741,#11739,#7346,.T.);
#15635=EDGE_CURVE('',#11740,#11741,#7347,.T.);
#15636=EDGE_CURVE('',#11742,#11740,#6082,.T.);
#15637=EDGE_CURVE('',#11743,#11741,#6083,.T.);
#15638=EDGE_CURVE('',#11742,#11743,#7348,.T.);
#15639=EDGE_CURVE('',#11744,#11742,#7349,.T.);
#15640=EDGE_CURVE('',#11745,#11743,#7350,.T.);
#15641=EDGE_CURVE('',#11744,#11745,#7351,.T.);
#15642=EDGE_CURVE('',#11746,#11744,#6084,.T.);
#15643=EDGE_CURVE('',#11747,#11745,#6085,.T.);
#15644=EDGE_CURVE('',#11746,#11747,#7352,.T.);
#15645=EDGE_CURVE('',#11748,#11746,#7353,.T.);
#15646=EDGE_CURVE('',#11749,#11747,#7354,.T.);
#15647=EDGE_CURVE('',#11748,#11749,#7355,.T.);
#15648=EDGE_CURVE('',#11750,#11748,#7356,.T.);
#15649=EDGE_CURVE('',#11751,#11749,#7357,.T.);
#15650=EDGE_CURVE('',#11750,#11751,#7358,.T.);
#15651=EDGE_CURVE('',#11752,#11750,#7359,.T.);
#15652=EDGE_CURVE('',#11753,#11751,#7360,.T.);
#15653=EDGE_CURVE('',#11752,#11753,#7361,.T.);
#15654=EDGE_CURVE('',#11752,#11754,#6086,.T.);
#15655=EDGE_CURVE('',#11755,#11753,#6087,.T.);
#15656=EDGE_CURVE('',#11754,#11755,#7362,.T.);
#15657=EDGE_CURVE('',#11756,#11754,#7363,.T.);
#15658=EDGE_CURVE('',#11757,#11755,#7364,.T.);
#15659=EDGE_CURVE('',#11756,#11757,#7365,.T.);
#15660=EDGE_CURVE('',#11758,#11756,#7366,.T.);
#15661=EDGE_CURVE('',#11759,#11757,#7367,.T.);
#15662=EDGE_CURVE('',#11758,#11759,#7368,.T.);
#15663=EDGE_CURVE('',#11707,#11758,#7369,.T.);
#15664=EDGE_CURVE('',#11708,#11759,#7370,.T.);
#21633=ORIENTED_EDGE('',*,*,#15178,.F.);
#21634=ORIENTED_EDGE('',*,*,#15179,.F.);
#21635=ORIENTED_EDGE('',*,*,#15180,.T.);
#21636=ORIENTED_EDGE('',*,*,#15181,.T.);
#21637=ORIENTED_EDGE('',*,*,#15180,.F.);
#21638=ORIENTED_EDGE('',*,*,#15181,.F.);
#21639=ORIENTED_EDGE('',*,*,#15182,.F.);
#21640=ORIENTED_EDGE('',*,*,#15183,.F.);
#21641=ORIENTED_EDGE('',*,*,#15184,.T.);
#21642=ORIENTED_EDGE('',*,*,#15185,.T.);
#21643=ORIENTED_EDGE('',*,*,#15184,.F.);
#21644=ORIENTED_EDGE('',*,*,#15185,.F.);
#21645=ORIENTED_EDGE('',*,*,#15178,.T.);
#21646=ORIENTED_EDGE('',*,*,#15186,.T.);
#21647=ORIENTED_EDGE('',*,*,#15182,.T.);
#21648=ORIENTED_EDGE('',*,*,#15187,.T.);
#21649=ORIENTED_EDGE('',*,*,#15188,.F.);
#21650=ORIENTED_EDGE('',*,*,#15189,.F.);
#21651=ORIENTED_EDGE('',*,*,#15190,.T.);
#21652=ORIENTED_EDGE('',*,*,#15191,.T.);
#21653=ORIENTED_EDGE('',*,*,#15192,.F.);
#21654=ORIENTED_EDGE('',*,*,#15193,.F.);
#21655=ORIENTED_EDGE('',*,*,#15194,.F.);
#21656=ORIENTED_EDGE('',*,*,#15195,.T.);
#21657=ORIENTED_EDGE('',*,*,#15196,.F.);
#21658=ORIENTED_EDGE('',*,*,#15197,.F.);
#21659=ORIENTED_EDGE('',*,*,#15198,.F.);
#21660=ORIENTED_EDGE('',*,*,#15199,.F.);
#21661=ORIENTED_EDGE('',*,*,#15200,.F.);
#21662=ORIENTED_EDGE('',*,*,#15201,.F.);
#21663=ORIENTED_EDGE('',*,*,#15202,.F.);
#21664=ORIENTED_EDGE('',*,*,#15203,.F.);
#21665=ORIENTED_EDGE('',*,*,#15204,.F.);
#21666=ORIENTED_EDGE('',*,*,#15205,.F.);
#21667=ORIENTED_EDGE('',*,*,#15206,.F.);
#21668=ORIENTED_EDGE('',*,*,#15207,.F.);
#21669=ORIENTED_EDGE('',*,*,#15208,.F.);
#21670=ORIENTED_EDGE('',*,*,#15209,.F.);
#21671=ORIENTED_EDGE('',*,*,#15210,.F.);
#21672=ORIENTED_EDGE('',*,*,#15211,.F.);
#21673=ORIENTED_EDGE('',*,*,#15212,.F.);
#21674=ORIENTED_EDGE('',*,*,#15213,.F.);
#21675=ORIENTED_EDGE('',*,*,#15214,.F.);
#21676=ORIENTED_EDGE('',*,*,#15215,.F.);
#21677=ORIENTED_EDGE('',*,*,#15216,.T.);
#21678=ORIENTED_EDGE('',*,*,#15217,.F.);
#21679=ORIENTED_EDGE('',*,*,#15218,.F.);
#21680=ORIENTED_EDGE('',*,*,#15219,.F.);
#21681=ORIENTED_EDGE('',*,*,#15220,.F.);
#21682=ORIENTED_EDGE('',*,*,#15221,.F.);
#21683=ORIENTED_EDGE('',*,*,#15222,.F.);
#21684=ORIENTED_EDGE('',*,*,#15223,.F.);
#21685=ORIENTED_EDGE('',*,*,#15224,.F.);
#21686=ORIENTED_EDGE('',*,*,#15225,.F.);
#21687=ORIENTED_EDGE('',*,*,#15226,.F.);
#21688=ORIENTED_EDGE('',*,*,#15227,.F.);
#21689=ORIENTED_EDGE('',*,*,#15228,.F.);
#21690=ORIENTED_EDGE('',*,*,#15229,.F.);
#21691=ORIENTED_EDGE('',*,*,#15230,.F.);
#21692=ORIENTED_EDGE('',*,*,#15231,.F.);
#21693=ORIENTED_EDGE('',*,*,#15232,.F.);
#21694=ORIENTED_EDGE('',*,*,#15233,.F.);
#21695=ORIENTED_EDGE('',*,*,#15234,.F.);
#21696=ORIENTED_EDGE('',*,*,#15235,.F.);
#21697=ORIENTED_EDGE('',*,*,#15236,.F.);
#21698=ORIENTED_EDGE('',*,*,#15237,.T.);
#21699=ORIENTED_EDGE('',*,*,#15238,.F.);
#21700=ORIENTED_EDGE('',*,*,#15193,.T.);
#21701=ORIENTED_EDGE('',*,*,#15239,.F.);
#21702=ORIENTED_EDGE('',*,*,#15237,.F.);
#21703=ORIENTED_EDGE('',*,*,#15240,.F.);
#21704=ORIENTED_EDGE('',*,*,#15241,.F.);
#21705=ORIENTED_EDGE('',*,*,#15242,.F.);
#21706=ORIENTED_EDGE('',*,*,#15243,.F.);
#21707=ORIENTED_EDGE('',*,*,#15244,.F.);
#21708=ORIENTED_EDGE('',*,*,#15245,.F.);
#21709=ORIENTED_EDGE('',*,*,#15216,.F.);
#21710=ORIENTED_EDGE('',*,*,#15246,.F.);
#21711=ORIENTED_EDGE('',*,*,#15247,.F.);
#21712=ORIENTED_EDGE('',*,*,#15248,.F.);
#21713=ORIENTED_EDGE('',*,*,#15249,.F.);
#21714=ORIENTED_EDGE('',*,*,#15250,.F.);
#21715=ORIENTED_EDGE('',*,*,#15251,.F.);
#21716=ORIENTED_EDGE('',*,*,#15195,.F.);
#21717=ORIENTED_EDGE('',*,*,#15252,.F.);
#21718=ORIENTED_EDGE('',*,*,#15253,.F.);
#21719=ORIENTED_EDGE('',*,*,#15254,.F.);
#21720=ORIENTED_EDGE('',*,*,#15255,.T.);
#21721=ORIENTED_EDGE('',*,*,#15256,.F.);
#21722=ORIENTED_EDGE('',*,*,#15257,.F.);
#21723=ORIENTED_EDGE('',*,*,#15258,.F.);
#21724=ORIENTED_EDGE('',*,*,#15259,.F.);
#21725=ORIENTED_EDGE('',*,*,#15260,.F.);
#21726=ORIENTED_EDGE('',*,*,#15261,.F.);
#21727=ORIENTED_EDGE('',*,*,#15262,.F.);
#21728=ORIENTED_EDGE('',*,*,#15263,.F.);
#21729=ORIENTED_EDGE('',*,*,#15264,.F.);
#21730=ORIENTED_EDGE('',*,*,#15265,.F.);
#21731=ORIENTED_EDGE('',*,*,#15266,.F.);
#21732=ORIENTED_EDGE('',*,*,#15267,.F.);
#21733=ORIENTED_EDGE('',*,*,#15268,.F.);
#21734=ORIENTED_EDGE('',*,*,#15269,.F.);
#21735=ORIENTED_EDGE('',*,*,#15270,.F.);
#21736=ORIENTED_EDGE('',*,*,#15271,.F.);
#21737=ORIENTED_EDGE('',*,*,#15272,.F.);
#21738=ORIENTED_EDGE('',*,*,#15273,.F.);
#21739=ORIENTED_EDGE('',*,*,#15274,.F.);
#21740=ORIENTED_EDGE('',*,*,#15275,.F.);
#21741=ORIENTED_EDGE('',*,*,#15276,.T.);
#21742=ORIENTED_EDGE('',*,*,#15277,.F.);
#21743=ORIENTED_EDGE('',*,*,#15278,.F.);
#21744=ORIENTED_EDGE('',*,*,#15279,.F.);
#21745=ORIENTED_EDGE('',*,*,#15280,.F.);
#21746=ORIENTED_EDGE('',*,*,#15281,.F.);
#21747=ORIENTED_EDGE('',*,*,#15282,.F.);
#21748=ORIENTED_EDGE('',*,*,#15283,.F.);
#21749=ORIENTED_EDGE('',*,*,#15284,.F.);
#21750=ORIENTED_EDGE('',*,*,#15285,.F.);
#21751=ORIENTED_EDGE('',*,*,#15286,.F.);
#21752=ORIENTED_EDGE('',*,*,#15287,.F.);
#21753=ORIENTED_EDGE('',*,*,#15288,.F.);
#21754=ORIENTED_EDGE('',*,*,#15289,.F.);
#21755=ORIENTED_EDGE('',*,*,#15290,.F.);
#21756=ORIENTED_EDGE('',*,*,#15291,.F.);
#21757=ORIENTED_EDGE('',*,*,#15292,.F.);
#21758=ORIENTED_EDGE('',*,*,#15293,.F.);
#21759=ORIENTED_EDGE('',*,*,#15294,.F.);
#21760=ORIENTED_EDGE('',*,*,#15295,.F.);
#21761=ORIENTED_EDGE('',*,*,#15296,.F.);
#21762=ORIENTED_EDGE('',*,*,#15297,.T.);
#21763=ORIENTED_EDGE('',*,*,#15298,.F.);
#21764=ORIENTED_EDGE('',*,*,#15253,.T.);
#21765=ORIENTED_EDGE('',*,*,#15299,.F.);
#21766=ORIENTED_EDGE('',*,*,#15297,.F.);
#21767=ORIENTED_EDGE('',*,*,#15300,.F.);
#21768=ORIENTED_EDGE('',*,*,#15301,.F.);
#21769=ORIENTED_EDGE('',*,*,#15302,.F.);
#21770=ORIENTED_EDGE('',*,*,#15303,.F.);
#21771=ORIENTED_EDGE('',*,*,#15304,.F.);
#21772=ORIENTED_EDGE('',*,*,#15305,.F.);
#21773=ORIENTED_EDGE('',*,*,#15276,.F.);
#21774=ORIENTED_EDGE('',*,*,#15306,.F.);
#21775=ORIENTED_EDGE('',*,*,#15307,.F.);
#21776=ORIENTED_EDGE('',*,*,#15308,.F.);
#21777=ORIENTED_EDGE('',*,*,#15309,.F.);
#21778=ORIENTED_EDGE('',*,*,#15310,.F.);
#21779=ORIENTED_EDGE('',*,*,#15311,.F.);
#21780=ORIENTED_EDGE('',*,*,#15255,.F.);
#21781=ORIENTED_EDGE('',*,*,#15312,.F.);
#21782=ORIENTED_EDGE('',*,*,#15313,.F.);
#21783=ORIENTED_EDGE('',*,*,#15314,.F.);
#21784=ORIENTED_EDGE('',*,*,#15315,.T.);
#21785=ORIENTED_EDGE('',*,*,#15316,.F.);
#21786=ORIENTED_EDGE('',*,*,#15317,.F.);
#21787=ORIENTED_EDGE('',*,*,#15318,.F.);
#21788=ORIENTED_EDGE('',*,*,#15319,.F.);
#21789=ORIENTED_EDGE('',*,*,#15320,.F.);
#21790=ORIENTED_EDGE('',*,*,#15321,.F.);
#21791=ORIENTED_EDGE('',*,*,#15322,.F.);
#21792=ORIENTED_EDGE('',*,*,#15323,.F.);
#21793=ORIENTED_EDGE('',*,*,#15324,.F.);
#21794=ORIENTED_EDGE('',*,*,#15325,.F.);
#21795=ORIENTED_EDGE('',*,*,#15326,.F.);
#21796=ORIENTED_EDGE('',*,*,#15327,.F.);
#21797=ORIENTED_EDGE('',*,*,#15328,.F.);
#21798=ORIENTED_EDGE('',*,*,#15329,.F.);
#21799=ORIENTED_EDGE('',*,*,#15330,.F.);
#21800=ORIENTED_EDGE('',*,*,#15331,.F.);
#21801=ORIENTED_EDGE('',*,*,#15332,.F.);
#21802=ORIENTED_EDGE('',*,*,#15333,.F.);
#21803=ORIENTED_EDGE('',*,*,#15334,.F.);
#21804=ORIENTED_EDGE('',*,*,#15335,.F.);
#21805=ORIENTED_EDGE('',*,*,#15336,.T.);
#21806=ORIENTED_EDGE('',*,*,#15337,.F.);
#21807=ORIENTED_EDGE('',*,*,#15338,.F.);
#21808=ORIENTED_EDGE('',*,*,#15339,.F.);
#21809=ORIENTED_EDGE('',*,*,#15340,.F.);
#21810=ORIENTED_EDGE('',*,*,#15341,.F.);
#21811=ORIENTED_EDGE('',*,*,#15342,.F.);
#21812=ORIENTED_EDGE('',*,*,#15343,.F.);
#21813=ORIENTED_EDGE('',*,*,#15344,.F.);
#21814=ORIENTED_EDGE('',*,*,#15345,.F.);
#21815=ORIENTED_EDGE('',*,*,#15346,.F.);
#21816=ORIENTED_EDGE('',*,*,#15347,.F.);
#21817=ORIENTED_EDGE('',*,*,#15348,.F.);
#21818=ORIENTED_EDGE('',*,*,#15349,.F.);
#21819=ORIENTED_EDGE('',*,*,#15350,.F.);
#21820=ORIENTED_EDGE('',*,*,#15351,.F.);
#21821=ORIENTED_EDGE('',*,*,#15352,.F.);
#21822=ORIENTED_EDGE('',*,*,#15353,.F.);
#21823=ORIENTED_EDGE('',*,*,#15354,.F.);
#21824=ORIENTED_EDGE('',*,*,#15355,.F.);
#21825=ORIENTED_EDGE('',*,*,#15356,.F.);
#21826=ORIENTED_EDGE('',*,*,#15357,.T.);
#21827=ORIENTED_EDGE('',*,*,#15358,.F.);
#21828=ORIENTED_EDGE('',*,*,#15313,.T.);
#21829=ORIENTED_EDGE('',*,*,#15359,.F.);
#21830=ORIENTED_EDGE('',*,*,#15357,.F.);
#21831=ORIENTED_EDGE('',*,*,#15360,.F.);
#21832=ORIENTED_EDGE('',*,*,#15361,.F.);
#21833=ORIENTED_EDGE('',*,*,#15362,.F.);
#21834=ORIENTED_EDGE('',*,*,#15363,.F.);
#21835=ORIENTED_EDGE('',*,*,#15364,.F.);
#21836=ORIENTED_EDGE('',*,*,#15365,.F.);
#21837=ORIENTED_EDGE('',*,*,#15336,.F.);
#21838=ORIENTED_EDGE('',*,*,#15366,.F.);
#21839=ORIENTED_EDGE('',*,*,#15367,.F.);
#21840=ORIENTED_EDGE('',*,*,#15368,.F.);
#21841=ORIENTED_EDGE('',*,*,#15369,.F.);
#21842=ORIENTED_EDGE('',*,*,#15370,.F.);
#21843=ORIENTED_EDGE('',*,*,#15371,.F.);
#21844=ORIENTED_EDGE('',*,*,#15315,.F.);
#21845=ORIENTED_EDGE('',*,*,#15200,.T.);
#21846=ORIENTED_EDGE('',*,*,#15372,.F.);
#21847=ORIENTED_EDGE('',*,*,#15373,.F.);
#21848=ORIENTED_EDGE('',*,*,#15374,.T.);
#21849=ORIENTED_EDGE('',*,*,#15375,.T.);
#21850=ORIENTED_EDGE('',*,*,#15376,.F.);
#21851=ORIENTED_EDGE('',*,*,#15320,.T.);
#21852=ORIENTED_EDGE('',*,*,#15377,.F.);
#21853=ORIENTED_EDGE('',*,*,#15260,.T.);
#21854=ORIENTED_EDGE('',*,*,#15378,.F.);
#21855=ORIENTED_EDGE('',*,*,#15199,.T.);
#21856=ORIENTED_EDGE('',*,*,#15379,.F.);
#21857=ORIENTED_EDGE('',*,*,#15380,.F.);
#21858=ORIENTED_EDGE('',*,*,#15372,.T.);
#21859=ORIENTED_EDGE('',*,*,#15321,.T.);
#21860=ORIENTED_EDGE('',*,*,#15376,.T.);
#21861=ORIENTED_EDGE('',*,*,#15381,.T.);
#21862=ORIENTED_EDGE('',*,*,#15382,.F.);
#21863=ORIENTED_EDGE('',*,*,#15261,.T.);
#21864=ORIENTED_EDGE('',*,*,#15377,.T.);
#21865=ORIENTED_EDGE('',*,*,#15319,.T.);
#21866=ORIENTED_EDGE('',*,*,#15383,.F.);
#21867=ORIENTED_EDGE('',*,*,#15198,.T.);
#21868=ORIENTED_EDGE('',*,*,#15384,.F.);
#21869=ORIENTED_EDGE('',*,*,#15385,.T.);
#21870=ORIENTED_EDGE('',*,*,#15379,.T.);
#21871=ORIENTED_EDGE('',*,*,#15322,.T.);
#21872=ORIENTED_EDGE('',*,*,#15382,.T.);
#21873=ORIENTED_EDGE('',*,*,#15386,.T.);
#21874=ORIENTED_EDGE('',*,*,#15387,.F.);
#21875=ORIENTED_EDGE('',*,*,#15262,.T.);
#21876=ORIENTED_EDGE('',*,*,#15383,.T.);
#21877=ORIENTED_EDGE('',*,*,#15318,.T.);
#21878=ORIENTED_EDGE('',*,*,#15388,.F.);
#21879=ORIENTED_EDGE('',*,*,#15197,.T.);
#21880=ORIENTED_EDGE('',*,*,#15389,.F.);
#21881=ORIENTED_EDGE('',*,*,#15390,.F.);
#21882=ORIENTED_EDGE('',*,*,#15384,.T.);
#21883=ORIENTED_EDGE('',*,*,#15323,.T.);
#21884=ORIENTED_EDGE('',*,*,#15387,.T.);
#21885=ORIENTED_EDGE('',*,*,#15391,.T.);
#21886=ORIENTED_EDGE('',*,*,#15392,.F.);
#21887=ORIENTED_EDGE('',*,*,#15263,.T.);
#21888=ORIENTED_EDGE('',*,*,#15388,.T.);
#21889=ORIENTED_EDGE('',*,*,#15317,.T.);
#21890=ORIENTED_EDGE('',*,*,#15393,.F.);
#21891=ORIENTED_EDGE('',*,*,#15196,.T.);
#21892=ORIENTED_EDGE('',*,*,#15251,.T.);
#21893=ORIENTED_EDGE('',*,*,#15394,.F.);
#21894=ORIENTED_EDGE('',*,*,#15395,.T.);
#21895=ORIENTED_EDGE('',*,*,#15389,.T.);
#21896=ORIENTED_EDGE('',*,*,#15324,.T.);
#21897=ORIENTED_EDGE('',*,*,#15392,.T.);
#21898=ORIENTED_EDGE('',*,*,#15396,.T.);
#21899=ORIENTED_EDGE('',*,*,#15397,.F.);
#21900=ORIENTED_EDGE('',*,*,#15264,.T.);
#21901=ORIENTED_EDGE('',*,*,#15393,.T.);
#21902=ORIENTED_EDGE('',*,*,#15316,.T.);
#21903=ORIENTED_EDGE('',*,*,#15371,.T.);
#21904=ORIENTED_EDGE('',*,*,#15398,.F.);
#21905=ORIENTED_EDGE('',*,*,#15250,.T.);
#21906=ORIENTED_EDGE('',*,*,#15399,.F.);
#21907=ORIENTED_EDGE('',*,*,#15400,.F.);
#21908=ORIENTED_EDGE('',*,*,#15394,.T.);
#21909=ORIENTED_EDGE('',*,*,#15325,.T.);
#21910=ORIENTED_EDGE('',*,*,#15397,.T.);
#21911=ORIENTED_EDGE('',*,*,#15401,.T.);
#21912=ORIENTED_EDGE('',*,*,#15402,.F.);
#21913=ORIENTED_EDGE('',*,*,#15265,.T.);
#21914=ORIENTED_EDGE('',*,*,#15398,.T.);
#21915=ORIENTED_EDGE('',*,*,#15370,.T.);
#21916=ORIENTED_EDGE('',*,*,#15403,.F.);
#21917=ORIENTED_EDGE('',*,*,#15249,.T.);
#21918=ORIENTED_EDGE('',*,*,#15404,.F.);
#21919=ORIENTED_EDGE('',*,*,#15405,.T.);
#21920=ORIENTED_EDGE('',*,*,#15399,.T.);
#21921=ORIENTED_EDGE('',*,*,#15326,.T.);
#21922=ORIENTED_EDGE('',*,*,#15402,.T.);
#21923=ORIENTED_EDGE('',*,*,#15406,.T.);
#21924=ORIENTED_EDGE('',*,*,#15407,.F.);
#21925=ORIENTED_EDGE('',*,*,#15266,.T.);
#21926=ORIENTED_EDGE('',*,*,#15403,.T.);
#21927=ORIENTED_EDGE('',*,*,#15369,.T.);
#21928=ORIENTED_EDGE('',*,*,#15408,.F.);
#21929=ORIENTED_EDGE('',*,*,#15248,.T.);
#21930=ORIENTED_EDGE('',*,*,#15409,.F.);
#21931=ORIENTED_EDGE('',*,*,#15410,.F.);
#21932=ORIENTED_EDGE('',*,*,#15404,.T.);
#21933=ORIENTED_EDGE('',*,*,#15327,.T.);
#21934=ORIENTED_EDGE('',*,*,#15407,.T.);
#21935=ORIENTED_EDGE('',*,*,#15411,.T.);
#21936=ORIENTED_EDGE('',*,*,#15412,.F.);
#21937=ORIENTED_EDGE('',*,*,#15267,.T.);
#21938=ORIENTED_EDGE('',*,*,#15408,.T.);
#21939=ORIENTED_EDGE('',*,*,#15368,.T.);
#21940=ORIENTED_EDGE('',*,*,#15413,.F.);
#21941=ORIENTED_EDGE('',*,*,#15247,.T.);
#21942=ORIENTED_EDGE('',*,*,#15414,.F.);
#21943=ORIENTED_EDGE('',*,*,#15415,.T.);
#21944=ORIENTED_EDGE('',*,*,#15409,.T.);
#21945=ORIENTED_EDGE('',*,*,#15328,.T.);
#21946=ORIENTED_EDGE('',*,*,#15412,.T.);
#21947=ORIENTED_EDGE('',*,*,#15416,.T.);
#21948=ORIENTED_EDGE('',*,*,#15417,.F.);
#21949=ORIENTED_EDGE('',*,*,#15268,.T.);
#21950=ORIENTED_EDGE('',*,*,#15413,.T.);
#21951=ORIENTED_EDGE('',*,*,#15367,.T.);
#21952=ORIENTED_EDGE('',*,*,#15418,.F.);
#21953=ORIENTED_EDGE('',*,*,#15246,.T.);
#21954=ORIENTED_EDGE('',*,*,#15215,.T.);
#21955=ORIENTED_EDGE('',*,*,#15419,.F.);
#21956=ORIENTED_EDGE('',*,*,#15420,.F.);
#21957=ORIENTED_EDGE('',*,*,#15414,.T.);
#21958=ORIENTED_EDGE('',*,*,#15329,.T.);
#21959=ORIENTED_EDGE('',*,*,#15417,.T.);
#21960=ORIENTED_EDGE('',*,*,#15421,.T.);
#21961=ORIENTED_EDGE('',*,*,#15422,.F.);
#21962=ORIENTED_EDGE('',*,*,#15269,.T.);
#21963=ORIENTED_EDGE('',*,*,#15418,.T.);
#21964=ORIENTED_EDGE('',*,*,#15366,.T.);
#21965=ORIENTED_EDGE('',*,*,#15335,.T.);
#21966=ORIENTED_EDGE('',*,*,#15423,.F.);
#21967=ORIENTED_EDGE('',*,*,#15214,.T.);
#21968=ORIENTED_EDGE('',*,*,#15424,.F.);
#21969=ORIENTED_EDGE('',*,*,#15425,.T.);
#21970=ORIENTED_EDGE('',*,*,#15419,.T.);
#21971=ORIENTED_EDGE('',*,*,#15330,.T.);
#21972=ORIENTED_EDGE('',*,*,#15422,.T.);
#21973=ORIENTED_EDGE('',*,*,#15426,.T.);
#21974=ORIENTED_EDGE('',*,*,#15427,.F.);
#21975=ORIENTED_EDGE('',*,*,#15270,.T.);
#21976=ORIENTED_EDGE('',*,*,#15423,.T.);
#21977=ORIENTED_EDGE('',*,*,#15334,.T.);
#21978=ORIENTED_EDGE('',*,*,#15428,.F.);
#21979=ORIENTED_EDGE('',*,*,#15213,.T.);
#21980=ORIENTED_EDGE('',*,*,#15429,.F.);
#21981=ORIENTED_EDGE('',*,*,#15430,.F.);
#21982=ORIENTED_EDGE('',*,*,#15424,.T.);
#21983=ORIENTED_EDGE('',*,*,#15331,.T.);
#21984=ORIENTED_EDGE('',*,*,#15427,.T.);
#21985=ORIENTED_EDGE('',*,*,#15431,.T.);
#21986=ORIENTED_EDGE('',*,*,#15432,.F.);
#21987=ORIENTED_EDGE('',*,*,#15271,.T.);
#21988=ORIENTED_EDGE('',*,*,#15428,.T.);
#21989=ORIENTED_EDGE('',*,*,#15333,.T.);
#21990=ORIENTED_EDGE('',*,*,#15433,.F.);
#21991=ORIENTED_EDGE('',*,*,#15232,.T.);
#21992=ORIENTED_EDGE('',*,*,#15434,.T.);
#21993=ORIENTED_EDGE('',*,*,#15292,.T.);
#21994=ORIENTED_EDGE('',*,*,#15435,.T.);
#21995=ORIENTED_EDGE('',*,*,#15352,.T.);
#21996=ORIENTED_EDGE('',*,*,#15436,.T.);
#21997=ORIENTED_EDGE('',*,*,#15437,.F.);
#21998=ORIENTED_EDGE('',*,*,#15438,.F.);
#21999=ORIENTED_EDGE('',*,*,#15439,.T.);
#22000=ORIENTED_EDGE('',*,*,#15440,.T.);
#22001=ORIENTED_EDGE('',*,*,#15351,.T.);
#22002=ORIENTED_EDGE('',*,*,#15441,.T.);
#22003=ORIENTED_EDGE('',*,*,#15442,.F.);
#22004=ORIENTED_EDGE('',*,*,#15436,.F.);
#22005=ORIENTED_EDGE('',*,*,#15291,.T.);
#22006=ORIENTED_EDGE('',*,*,#15443,.T.);
#22007=ORIENTED_EDGE('',*,*,#15353,.T.);
#22008=ORIENTED_EDGE('',*,*,#15435,.F.);
#22009=ORIENTED_EDGE('',*,*,#15231,.T.);
#22010=ORIENTED_EDGE('',*,*,#15444,.T.);
#22011=ORIENTED_EDGE('',*,*,#15293,.T.);
#22012=ORIENTED_EDGE('',*,*,#15434,.F.);
#22013=ORIENTED_EDGE('',*,*,#15350,.T.);
#22014=ORIENTED_EDGE('',*,*,#15445,.T.);
#22015=ORIENTED_EDGE('',*,*,#15446,.F.);
#22016=ORIENTED_EDGE('',*,*,#15441,.F.);
#22017=ORIENTED_EDGE('',*,*,#15290,.T.);
#22018=ORIENTED_EDGE('',*,*,#15447,.T.);
#22019=ORIENTED_EDGE('',*,*,#15354,.T.);
#22020=ORIENTED_EDGE('',*,*,#15443,.F.);
#22021=ORIENTED_EDGE('',*,*,#15230,.T.);
#22022=ORIENTED_EDGE('',*,*,#15448,.T.);
#22023=ORIENTED_EDGE('',*,*,#15294,.T.);
#22024=ORIENTED_EDGE('',*,*,#15444,.F.);
#22025=ORIENTED_EDGE('',*,*,#15349,.T.);
#22026=ORIENTED_EDGE('',*,*,#15449,.T.);
#22027=ORIENTED_EDGE('',*,*,#15450,.F.);
#22028=ORIENTED_EDGE('',*,*,#15445,.F.);
#22029=ORIENTED_EDGE('',*,*,#15289,.T.);
#22030=ORIENTED_EDGE('',*,*,#15451,.T.);
#22031=ORIENTED_EDGE('',*,*,#15355,.T.);
#22032=ORIENTED_EDGE('',*,*,#15447,.F.);
#22033=ORIENTED_EDGE('',*,*,#15229,.T.);
#22034=ORIENTED_EDGE('',*,*,#15452,.T.);
#22035=ORIENTED_EDGE('',*,*,#15295,.T.);
#22036=ORIENTED_EDGE('',*,*,#15448,.F.);
#22037=ORIENTED_EDGE('',*,*,#15348,.T.);
#22038=ORIENTED_EDGE('',*,*,#15453,.T.);
#22039=ORIENTED_EDGE('',*,*,#15454,.F.);
#22040=ORIENTED_EDGE('',*,*,#15449,.F.);
#22041=ORIENTED_EDGE('',*,*,#15288,.T.);
#22042=ORIENTED_EDGE('',*,*,#15455,.T.);
#22043=ORIENTED_EDGE('',*,*,#15360,.T.);
#22044=ORIENTED_EDGE('',*,*,#15356,.T.);
#22045=ORIENTED_EDGE('',*,*,#15451,.F.);
#22046=ORIENTED_EDGE('',*,*,#15228,.T.);
#22047=ORIENTED_EDGE('',*,*,#15456,.T.);
#22048=ORIENTED_EDGE('',*,*,#15300,.T.);
#22049=ORIENTED_EDGE('',*,*,#15296,.T.);
#22050=ORIENTED_EDGE('',*,*,#15452,.F.);
#22051=ORIENTED_EDGE('',*,*,#15347,.T.);
#22052=ORIENTED_EDGE('',*,*,#15457,.T.);
#22053=ORIENTED_EDGE('',*,*,#15458,.F.);
#22054=ORIENTED_EDGE('',*,*,#15453,.F.);
#22055=ORIENTED_EDGE('',*,*,#15287,.T.);
#22056=ORIENTED_EDGE('',*,*,#15459,.T.);
#22057=ORIENTED_EDGE('',*,*,#15361,.T.);
#22058=ORIENTED_EDGE('',*,*,#15455,.F.);
#22059=ORIENTED_EDGE('',*,*,#15227,.T.);
#22060=ORIENTED_EDGE('',*,*,#15460,.T.);
#22061=ORIENTED_EDGE('',*,*,#15301,.T.);
#22062=ORIENTED_EDGE('',*,*,#15456,.F.);
#22063=ORIENTED_EDGE('',*,*,#15346,.T.);
#22064=ORIENTED_EDGE('',*,*,#15461,.T.);
#22065=ORIENTED_EDGE('',*,*,#15462,.F.);
#22066=ORIENTED_EDGE('',*,*,#15457,.F.);
#22067=ORIENTED_EDGE('',*,*,#15286,.T.);
#22068=ORIENTED_EDGE('',*,*,#15463,.T.);
#22069=ORIENTED_EDGE('',*,*,#15362,.T.);
#22070=ORIENTED_EDGE('',*,*,#15459,.F.);
#22071=ORIENTED_EDGE('',*,*,#15226,.T.);
#22072=ORIENTED_EDGE('',*,*,#15464,.T.);
#22073=ORIENTED_EDGE('',*,*,#15302,.T.);
#22074=ORIENTED_EDGE('',*,*,#15460,.F.);
#22075=ORIENTED_EDGE('',*,*,#15345,.T.);
#22076=ORIENTED_EDGE('',*,*,#15465,.T.);
#22077=ORIENTED_EDGE('',*,*,#15466,.F.);
#22078=ORIENTED_EDGE('',*,*,#15461,.F.);
#22079=ORIENTED_EDGE('',*,*,#15285,.T.);
#22080=ORIENTED_EDGE('',*,*,#15467,.T.);
#22081=ORIENTED_EDGE('',*,*,#15363,.T.);
#22082=ORIENTED_EDGE('',*,*,#15463,.F.);
#22083=ORIENTED_EDGE('',*,*,#15225,.T.);
#22084=ORIENTED_EDGE('',*,*,#15468,.T.);
#22085=ORIENTED_EDGE('',*,*,#15303,.T.);
#22086=ORIENTED_EDGE('',*,*,#15464,.F.);
#22087=ORIENTED_EDGE('',*,*,#15344,.T.);
#22088=ORIENTED_EDGE('',*,*,#15469,.T.);
#22089=ORIENTED_EDGE('',*,*,#15470,.F.);
#22090=ORIENTED_EDGE('',*,*,#15465,.F.);
#22091=ORIENTED_EDGE('',*,*,#15284,.T.);
#22092=ORIENTED_EDGE('',*,*,#15471,.T.);
#22093=ORIENTED_EDGE('',*,*,#15364,.T.);
#22094=ORIENTED_EDGE('',*,*,#15467,.F.);
#22095=ORIENTED_EDGE('',*,*,#15224,.T.);
#22096=ORIENTED_EDGE('',*,*,#15472,.T.);
#22097=ORIENTED_EDGE('',*,*,#15304,.T.);
#22098=ORIENTED_EDGE('',*,*,#15468,.F.);
#22099=ORIENTED_EDGE('',*,*,#15343,.T.);
#22100=ORIENTED_EDGE('',*,*,#15473,.T.);
#22101=ORIENTED_EDGE('',*,*,#15474,.F.);
#22102=ORIENTED_EDGE('',*,*,#15469,.F.);
#22103=ORIENTED_EDGE('',*,*,#15283,.T.);
#22104=ORIENTED_EDGE('',*,*,#15475,.T.);
#22105=ORIENTED_EDGE('',*,*,#15337,.T.);
#22106=ORIENTED_EDGE('',*,*,#15365,.T.);
#22107=ORIENTED_EDGE('',*,*,#15471,.F.);
#22108=ORIENTED_EDGE('',*,*,#15223,.T.);
#22109=ORIENTED_EDGE('',*,*,#15476,.T.);
#22110=ORIENTED_EDGE('',*,*,#15277,.T.);
#22111=ORIENTED_EDGE('',*,*,#15305,.T.);
#22112=ORIENTED_EDGE('',*,*,#15472,.F.);
#22113=ORIENTED_EDGE('',*,*,#15342,.T.);
#22114=ORIENTED_EDGE('',*,*,#15477,.T.);
#22115=ORIENTED_EDGE('',*,*,#15478,.F.);
#22116=ORIENTED_EDGE('',*,*,#15473,.F.);
#22117=ORIENTED_EDGE('',*,*,#15282,.T.);
#22118=ORIENTED_EDGE('',*,*,#15479,.T.);
#22119=ORIENTED_EDGE('',*,*,#15338,.T.);
#22120=ORIENTED_EDGE('',*,*,#15475,.F.);
#22121=ORIENTED_EDGE('',*,*,#15222,.T.);
#22122=ORIENTED_EDGE('',*,*,#15480,.T.);
#22123=ORIENTED_EDGE('',*,*,#15278,.T.);
#22124=ORIENTED_EDGE('',*,*,#15476,.F.);
#22125=ORIENTED_EDGE('',*,*,#15341,.T.);
#22126=ORIENTED_EDGE('',*,*,#15481,.T.);
#22127=ORIENTED_EDGE('',*,*,#15482,.F.);
#22128=ORIENTED_EDGE('',*,*,#15477,.F.);
#22129=ORIENTED_EDGE('',*,*,#15281,.T.);
#22130=ORIENTED_EDGE('',*,*,#15483,.T.);
#22131=ORIENTED_EDGE('',*,*,#15339,.T.);
#22132=ORIENTED_EDGE('',*,*,#15479,.F.);
#22133=ORIENTED_EDGE('',*,*,#15221,.T.);
#22134=ORIENTED_EDGE('',*,*,#15484,.T.);
#22135=ORIENTED_EDGE('',*,*,#15279,.T.);
#22136=ORIENTED_EDGE('',*,*,#15480,.F.);
#22137=ORIENTED_EDGE('',*,*,#15485,.F.);
#22138=ORIENTED_EDGE('',*,*,#15486,.T.);
#22139=ORIENTED_EDGE('',*,*,#15487,.F.);
#22140=ORIENTED_EDGE('',*,*,#15486,.F.);
#22141=ORIENTED_EDGE('',*,*,#15488,.F.);
#22142=ORIENTED_EDGE('',*,*,#15489,.T.);
#22143=ORIENTED_EDGE('',*,*,#15490,.F.);
#22144=ORIENTED_EDGE('',*,*,#15489,.F.);
#22145=ORIENTED_EDGE('',*,*,#15491,.F.);
#22146=ORIENTED_EDGE('',*,*,#15492,.T.);
#22147=ORIENTED_EDGE('',*,*,#15493,.F.);
#22148=ORIENTED_EDGE('',*,*,#15492,.F.);
#22149=ORIENTED_EDGE('',*,*,#15494,.T.);
#22150=ORIENTED_EDGE('',*,*,#15495,.T.);
#22151=ORIENTED_EDGE('',*,*,#15496,.T.);
#22152=ORIENTED_EDGE('',*,*,#15497,.F.);
#22153=ORIENTED_EDGE('',*,*,#15179,.T.);
#22154=ORIENTED_EDGE('',*,*,#15191,.F.);
#22155=ORIENTED_EDGE('',*,*,#15498,.F.);
#22156=ORIENTED_EDGE('',*,*,#15499,.T.);
#22157=ORIENTED_EDGE('',*,*,#15500,.T.);
#22158=ORIENTED_EDGE('',*,*,#15187,.F.);
#22159=ORIENTED_EDGE('',*,*,#15183,.T.);
#22160=ORIENTED_EDGE('',*,*,#15186,.F.);
#22161=ORIENTED_EDGE('',*,*,#15501,.F.);
#22162=ORIENTED_EDGE('',*,*,#15502,.T.);
#22163=ORIENTED_EDGE('',*,*,#15503,.T.);
#22164=ORIENTED_EDGE('',*,*,#15499,.F.);
#22165=ORIENTED_EDGE('',*,*,#15504,.F.);
#22166=ORIENTED_EDGE('',*,*,#15505,.T.);
#22167=ORIENTED_EDGE('',*,*,#15506,.T.);
#22168=ORIENTED_EDGE('',*,*,#15502,.F.);
#22169=ORIENTED_EDGE('',*,*,#15212,.T.);
#22170=ORIENTED_EDGE('',*,*,#15507,.T.);
#22171=ORIENTED_EDGE('',*,*,#15272,.T.);
#22172=ORIENTED_EDGE('',*,*,#15433,.T.);
#22173=ORIENTED_EDGE('',*,*,#15332,.T.);
#22174=ORIENTED_EDGE('',*,*,#15432,.T.);
#22175=ORIENTED_EDGE('',*,*,#15508,.T.);
#22176=ORIENTED_EDGE('',*,*,#15505,.F.);
#22177=ORIENTED_EDGE('',*,*,#15509,.F.);
#22178=ORIENTED_EDGE('',*,*,#15429,.T.);
#22179=ORIENTED_EDGE('',*,*,#15211,.T.);
#22180=ORIENTED_EDGE('',*,*,#15510,.T.);
#22181=ORIENTED_EDGE('',*,*,#15273,.T.);
#22182=ORIENTED_EDGE('',*,*,#15507,.F.);
#22183=ORIENTED_EDGE('',*,*,#15210,.T.);
#22184=ORIENTED_EDGE('',*,*,#15511,.T.);
#22185=ORIENTED_EDGE('',*,*,#15274,.T.);
#22186=ORIENTED_EDGE('',*,*,#15510,.F.);
#22187=ORIENTED_EDGE('',*,*,#15209,.T.);
#22188=ORIENTED_EDGE('',*,*,#15512,.T.);
#22189=ORIENTED_EDGE('',*,*,#15306,.T.);
#22190=ORIENTED_EDGE('',*,*,#15275,.T.);
#22191=ORIENTED_EDGE('',*,*,#15511,.F.);
#22192=ORIENTED_EDGE('',*,*,#15208,.T.);
#22193=ORIENTED_EDGE('',*,*,#15513,.T.);
#22194=ORIENTED_EDGE('',*,*,#15307,.T.);
#22195=ORIENTED_EDGE('',*,*,#15512,.F.);
#22196=ORIENTED_EDGE('',*,*,#15207,.T.);
#22197=ORIENTED_EDGE('',*,*,#15514,.T.);
#22198=ORIENTED_EDGE('',*,*,#15308,.T.);
#22199=ORIENTED_EDGE('',*,*,#15513,.F.);
#22200=ORIENTED_EDGE('',*,*,#15206,.T.);
#22201=ORIENTED_EDGE('',*,*,#15515,.T.);
#22202=ORIENTED_EDGE('',*,*,#15309,.T.);
#22203=ORIENTED_EDGE('',*,*,#15514,.F.);
#22204=ORIENTED_EDGE('',*,*,#15205,.T.);
#22205=ORIENTED_EDGE('',*,*,#15516,.T.);
#22206=ORIENTED_EDGE('',*,*,#15310,.T.);
#22207=ORIENTED_EDGE('',*,*,#15515,.F.);
#22208=ORIENTED_EDGE('',*,*,#15204,.T.);
#22209=ORIENTED_EDGE('',*,*,#15517,.T.);
#22210=ORIENTED_EDGE('',*,*,#15256,.T.);
#22211=ORIENTED_EDGE('',*,*,#15311,.T.);
#22212=ORIENTED_EDGE('',*,*,#15516,.F.);
#22213=ORIENTED_EDGE('',*,*,#15203,.T.);
#22214=ORIENTED_EDGE('',*,*,#15518,.T.);
#22215=ORIENTED_EDGE('',*,*,#15257,.T.);
#22216=ORIENTED_EDGE('',*,*,#15517,.F.);
#22217=ORIENTED_EDGE('',*,*,#15202,.T.);
#22218=ORIENTED_EDGE('',*,*,#15519,.T.);
#22219=ORIENTED_EDGE('',*,*,#15258,.T.);
#22220=ORIENTED_EDGE('',*,*,#15518,.F.);
#22221=ORIENTED_EDGE('',*,*,#15201,.T.);
#22222=ORIENTED_EDGE('',*,*,#15378,.T.);
#22223=ORIENTED_EDGE('',*,*,#15259,.T.);
#22224=ORIENTED_EDGE('',*,*,#15519,.F.);
#22225=ORIENTED_EDGE('',*,*,#15520,.F.);
#22226=ORIENTED_EDGE('',*,*,#15521,.T.);
#22227=ORIENTED_EDGE('',*,*,#15522,.T.);
#22228=ORIENTED_EDGE('',*,*,#15374,.F.);
#22229=ORIENTED_EDGE('',*,*,#15523,.F.);
#22230=ORIENTED_EDGE('',*,*,#15524,.T.);
#22231=ORIENTED_EDGE('',*,*,#15525,.T.);
#22232=ORIENTED_EDGE('',*,*,#15521,.F.);
#22233=ORIENTED_EDGE('',*,*,#15526,.F.);
#22234=ORIENTED_EDGE('',*,*,#15527,.T.);
#22235=ORIENTED_EDGE('',*,*,#15528,.T.);
#22236=ORIENTED_EDGE('',*,*,#15524,.F.);
#22237=ORIENTED_EDGE('',*,*,#15529,.F.);
#22238=ORIENTED_EDGE('',*,*,#15530,.T.);
#22239=ORIENTED_EDGE('',*,*,#15531,.T.);
#22240=ORIENTED_EDGE('',*,*,#15527,.F.);
#22241=ORIENTED_EDGE('',*,*,#15532,.F.);
#22242=ORIENTED_EDGE('',*,*,#15533,.T.);
#22243=ORIENTED_EDGE('',*,*,#15534,.T.);
#22244=ORIENTED_EDGE('',*,*,#15530,.F.);
#22245=ORIENTED_EDGE('',*,*,#15194,.T.);
#22246=ORIENTED_EDGE('',*,*,#15254,.T.);
#22247=ORIENTED_EDGE('',*,*,#15314,.T.);
#22248=ORIENTED_EDGE('',*,*,#15535,.T.);
#22249=ORIENTED_EDGE('',*,*,#15536,.T.);
#22250=ORIENTED_EDGE('',*,*,#15537,.T.);
#22251=ORIENTED_EDGE('',*,*,#15533,.F.);
#22252=ORIENTED_EDGE('',*,*,#15538,.F.);
#22253=ORIENTED_EDGE('',*,*,#15539,.T.);
#22254=ORIENTED_EDGE('',*,*,#15540,.T.);
#22255=ORIENTED_EDGE('',*,*,#15536,.F.);
#22256=ORIENTED_EDGE('',*,*,#15541,.F.);
#22257=ORIENTED_EDGE('',*,*,#15542,.T.);
#22258=ORIENTED_EDGE('',*,*,#15543,.T.);
#22259=ORIENTED_EDGE('',*,*,#15539,.F.);
#22260=ORIENTED_EDGE('',*,*,#15544,.F.);
#22261=ORIENTED_EDGE('',*,*,#15545,.T.);
#22262=ORIENTED_EDGE('',*,*,#15546,.T.);
#22263=ORIENTED_EDGE('',*,*,#15542,.F.);
#22264=ORIENTED_EDGE('',*,*,#15547,.F.);
#22265=ORIENTED_EDGE('',*,*,#15548,.T.);
#22266=ORIENTED_EDGE('',*,*,#15549,.T.);
#22267=ORIENTED_EDGE('',*,*,#15545,.F.);
#22268=ORIENTED_EDGE('',*,*,#15550,.F.);
#22269=ORIENTED_EDGE('',*,*,#15551,.T.);
#22270=ORIENTED_EDGE('',*,*,#15552,.T.);
#22271=ORIENTED_EDGE('',*,*,#15548,.F.);
#22272=ORIENTED_EDGE('',*,*,#15485,.T.);
#22273=ORIENTED_EDGE('',*,*,#15488,.T.);
#22274=ORIENTED_EDGE('',*,*,#15491,.T.);
#22275=ORIENTED_EDGE('',*,*,#15553,.F.);
#22276=ORIENTED_EDGE('',*,*,#15554,.T.);
#22277=ORIENTED_EDGE('',*,*,#15555,.T.);
#22278=ORIENTED_EDGE('',*,*,#15551,.F.);
#22279=ORIENTED_EDGE('',*,*,#15556,.F.);
#22280=ORIENTED_EDGE('',*,*,#15557,.T.);
#22281=ORIENTED_EDGE('',*,*,#15558,.T.);
#22282=ORIENTED_EDGE('',*,*,#15554,.F.);
#22283=ORIENTED_EDGE('',*,*,#15559,.F.);
#22284=ORIENTED_EDGE('',*,*,#15560,.T.);
#22285=ORIENTED_EDGE('',*,*,#15561,.T.);
#22286=ORIENTED_EDGE('',*,*,#15557,.F.);
#22287=ORIENTED_EDGE('',*,*,#15562,.F.);
#22288=ORIENTED_EDGE('',*,*,#15563,.T.);
#22289=ORIENTED_EDGE('',*,*,#15564,.T.);
#22290=ORIENTED_EDGE('',*,*,#15560,.F.);
#22291=ORIENTED_EDGE('',*,*,#15487,.T.);
#22292=ORIENTED_EDGE('',*,*,#15490,.T.);
#22293=ORIENTED_EDGE('',*,*,#15493,.T.);
#22294=ORIENTED_EDGE('',*,*,#15565,.T.);
#22295=ORIENTED_EDGE('',*,*,#15566,.T.);
#22296=ORIENTED_EDGE('',*,*,#15567,.T.);
#22297=ORIENTED_EDGE('',*,*,#15563,.F.);
#22298=ORIENTED_EDGE('',*,*,#15568,.F.);
#22299=ORIENTED_EDGE('',*,*,#15569,.T.);
#22300=ORIENTED_EDGE('',*,*,#15570,.T.);
#22301=ORIENTED_EDGE('',*,*,#15566,.F.);
#22302=ORIENTED_EDGE('',*,*,#15571,.F.);
#22303=ORIENTED_EDGE('',*,*,#15572,.T.);
#22304=ORIENTED_EDGE('',*,*,#15573,.T.);
#22305=ORIENTED_EDGE('',*,*,#15569,.F.);
#22306=ORIENTED_EDGE('',*,*,#15574,.F.);
#22307=ORIENTED_EDGE('',*,*,#15497,.T.);
#22308=ORIENTED_EDGE('',*,*,#15575,.T.);
#22309=ORIENTED_EDGE('',*,*,#15572,.F.);
#22310=ORIENTED_EDGE('',*,*,#15576,.F.);
#22311=ORIENTED_EDGE('',*,*,#15577,.T.);
#22312=ORIENTED_EDGE('',*,*,#15578,.F.);
#22313=ORIENTED_EDGE('',*,*,#15495,.F.);
#22314=ORIENTED_EDGE('',*,*,#15579,.T.);
#22315=ORIENTED_EDGE('',*,*,#15189,.T.);
#22316=ORIENTED_EDGE('',*,*,#15580,.F.);
#22317=ORIENTED_EDGE('',*,*,#15581,.F.);
#22318=ORIENTED_EDGE('',*,*,#15582,.T.);
#22319=ORIENTED_EDGE('',*,*,#15581,.T.);
#22320=ORIENTED_EDGE('',*,*,#15583,.F.);
#22321=ORIENTED_EDGE('',*,*,#15584,.F.);
#22322=ORIENTED_EDGE('',*,*,#15220,.T.);
#22323=ORIENTED_EDGE('',*,*,#15585,.F.);
#22324=ORIENTED_EDGE('',*,*,#15586,.T.);
#22325=ORIENTED_EDGE('',*,*,#15584,.T.);
#22326=ORIENTED_EDGE('',*,*,#15587,.F.);
#22327=ORIENTED_EDGE('',*,*,#15481,.F.);
#22328=ORIENTED_EDGE('',*,*,#15340,.T.);
#22329=ORIENTED_EDGE('',*,*,#15483,.F.);
#22330=ORIENTED_EDGE('',*,*,#15280,.T.);
#22331=ORIENTED_EDGE('',*,*,#15484,.F.);
#22332=ORIENTED_EDGE('',*,*,#15219,.T.);
#22333=ORIENTED_EDGE('',*,*,#15588,.F.);
#22334=ORIENTED_EDGE('',*,*,#15589,.T.);
#22335=ORIENTED_EDGE('',*,*,#15585,.T.);
#22336=ORIENTED_EDGE('',*,*,#15218,.T.);
#22337=ORIENTED_EDGE('',*,*,#15590,.F.);
#22338=ORIENTED_EDGE('',*,*,#15591,.F.);
#22339=ORIENTED_EDGE('',*,*,#15588,.T.);
#22340=ORIENTED_EDGE('',*,*,#15217,.T.);
#22341=ORIENTED_EDGE('',*,*,#15245,.T.);
#22342=ORIENTED_EDGE('',*,*,#15592,.F.);
#22343=ORIENTED_EDGE('',*,*,#15593,.T.);
#22344=ORIENTED_EDGE('',*,*,#15590,.T.);
#22345=ORIENTED_EDGE('',*,*,#15244,.T.);
#22346=ORIENTED_EDGE('',*,*,#15594,.F.);
#22347=ORIENTED_EDGE('',*,*,#15595,.F.);
#22348=ORIENTED_EDGE('',*,*,#15592,.T.);
#22349=ORIENTED_EDGE('',*,*,#15243,.T.);
#22350=ORIENTED_EDGE('',*,*,#15596,.F.);
#22351=ORIENTED_EDGE('',*,*,#15597,.T.);
#22352=ORIENTED_EDGE('',*,*,#15594,.T.);
#22353=ORIENTED_EDGE('',*,*,#15242,.T.);
#22354=ORIENTED_EDGE('',*,*,#15598,.F.);
#22355=ORIENTED_EDGE('',*,*,#15599,.F.);
#22356=ORIENTED_EDGE('',*,*,#15596,.T.);
#22357=ORIENTED_EDGE('',*,*,#15241,.T.);
#22358=ORIENTED_EDGE('',*,*,#15600,.F.);
#22359=ORIENTED_EDGE('',*,*,#15601,.T.);
#22360=ORIENTED_EDGE('',*,*,#15598,.T.);
#22361=ORIENTED_EDGE('',*,*,#15240,.T.);
#22362=ORIENTED_EDGE('',*,*,#15236,.T.);
#22363=ORIENTED_EDGE('',*,*,#15602,.F.);
#22364=ORIENTED_EDGE('',*,*,#15603,.F.);
#22365=ORIENTED_EDGE('',*,*,#15600,.T.);
#22366=ORIENTED_EDGE('',*,*,#15235,.T.);
#22367=ORIENTED_EDGE('',*,*,#15604,.F.);
#22368=ORIENTED_EDGE('',*,*,#15605,.T.);
#22369=ORIENTED_EDGE('',*,*,#15602,.T.);
#22370=ORIENTED_EDGE('',*,*,#15234,.T.);
#22371=ORIENTED_EDGE('',*,*,#15606,.F.);
#22372=ORIENTED_EDGE('',*,*,#15607,.F.);
#22373=ORIENTED_EDGE('',*,*,#15604,.T.);
#22374=ORIENTED_EDGE('',*,*,#15233,.T.);
#22375=ORIENTED_EDGE('',*,*,#15440,.F.);
#22376=ORIENTED_EDGE('',*,*,#15608,.T.);
#22377=ORIENTED_EDGE('',*,*,#15606,.T.);
#22378=ORIENTED_EDGE('',*,*,#15609,.T.);
#22379=ORIENTED_EDGE('',*,*,#15438,.T.);
#22380=ORIENTED_EDGE('',*,*,#15610,.F.);
#22381=ORIENTED_EDGE('',*,*,#15611,.F.);
#22382=ORIENTED_EDGE('',*,*,#15612,.T.);
#22383=ORIENTED_EDGE('',*,*,#15611,.T.);
#22384=ORIENTED_EDGE('',*,*,#15613,.F.);
#22385=ORIENTED_EDGE('',*,*,#15614,.F.);
#22386=ORIENTED_EDGE('',*,*,#15615,.T.);
#22387=ORIENTED_EDGE('',*,*,#15614,.T.);
#22388=ORIENTED_EDGE('',*,*,#15616,.F.);
#22389=ORIENTED_EDGE('',*,*,#15617,.F.);
#22390=ORIENTED_EDGE('',*,*,#15618,.T.);
#22391=ORIENTED_EDGE('',*,*,#15617,.T.);
#22392=ORIENTED_EDGE('',*,*,#15619,.F.);
#22393=ORIENTED_EDGE('',*,*,#15620,.F.);
#22394=ORIENTED_EDGE('',*,*,#15621,.T.);
#22395=ORIENTED_EDGE('',*,*,#15620,.T.);
#22396=ORIENTED_EDGE('',*,*,#15622,.F.);
#22397=ORIENTED_EDGE('',*,*,#15623,.F.);
#22398=ORIENTED_EDGE('',*,*,#15238,.T.);
#22399=ORIENTED_EDGE('',*,*,#15239,.T.);
#22400=ORIENTED_EDGE('',*,*,#15192,.T.);
#22401=ORIENTED_EDGE('',*,*,#15298,.T.);
#22402=ORIENTED_EDGE('',*,*,#15299,.T.);
#22403=ORIENTED_EDGE('',*,*,#15252,.T.);
#22404=ORIENTED_EDGE('',*,*,#15358,.T.);
#22405=ORIENTED_EDGE('',*,*,#15359,.T.);
#22406=ORIENTED_EDGE('',*,*,#15312,.T.);
#22407=ORIENTED_EDGE('',*,*,#15624,.F.);
#22408=ORIENTED_EDGE('',*,*,#15623,.T.);
#22409=ORIENTED_EDGE('',*,*,#15625,.F.);
#22410=ORIENTED_EDGE('',*,*,#15626,.F.);
#22411=ORIENTED_EDGE('',*,*,#15627,.T.);
#22412=ORIENTED_EDGE('',*,*,#15626,.T.);
#22413=ORIENTED_EDGE('',*,*,#15628,.F.);
#22414=ORIENTED_EDGE('',*,*,#15629,.F.);
#22415=ORIENTED_EDGE('',*,*,#15630,.T.);
#22416=ORIENTED_EDGE('',*,*,#15629,.T.);
#22417=ORIENTED_EDGE('',*,*,#15631,.F.);
#22418=ORIENTED_EDGE('',*,*,#15632,.F.);
#22419=ORIENTED_EDGE('',*,*,#15633,.T.);
#22420=ORIENTED_EDGE('',*,*,#15632,.T.);
#22421=ORIENTED_EDGE('',*,*,#15634,.F.);
#22422=ORIENTED_EDGE('',*,*,#15635,.F.);
#22423=ORIENTED_EDGE('',*,*,#15636,.T.);
#22424=ORIENTED_EDGE('',*,*,#15635,.T.);
#22425=ORIENTED_EDGE('',*,*,#15637,.F.);
#22426=ORIENTED_EDGE('',*,*,#15638,.F.);
#22427=ORIENTED_EDGE('',*,*,#15639,.T.);
#22428=ORIENTED_EDGE('',*,*,#15638,.T.);
#22429=ORIENTED_EDGE('',*,*,#15640,.F.);
#22430=ORIENTED_EDGE('',*,*,#15641,.F.);
#22431=ORIENTED_EDGE('',*,*,#15642,.T.);
#22432=ORIENTED_EDGE('',*,*,#15641,.T.);
#22433=ORIENTED_EDGE('',*,*,#15643,.F.);
#22434=ORIENTED_EDGE('',*,*,#15644,.F.);
#22435=ORIENTED_EDGE('',*,*,#15645,.T.);
#22436=ORIENTED_EDGE('',*,*,#15644,.T.);
#22437=ORIENTED_EDGE('',*,*,#15646,.F.);
#22438=ORIENTED_EDGE('',*,*,#15647,.F.);
#22439=ORIENTED_EDGE('',*,*,#15648,.T.);
#22440=ORIENTED_EDGE('',*,*,#15647,.T.);
#22441=ORIENTED_EDGE('',*,*,#15649,.F.);
#22442=ORIENTED_EDGE('',*,*,#15650,.F.);
#22443=ORIENTED_EDGE('',*,*,#15651,.T.);
#22444=ORIENTED_EDGE('',*,*,#15650,.T.);
#22445=ORIENTED_EDGE('',*,*,#15652,.F.);
#22446=ORIENTED_EDGE('',*,*,#15653,.F.);
#22447=ORIENTED_EDGE('',*,*,#15654,.F.);
#22448=ORIENTED_EDGE('',*,*,#15653,.T.);
#22449=ORIENTED_EDGE('',*,*,#15655,.F.);
#22450=ORIENTED_EDGE('',*,*,#15656,.F.);
#22451=ORIENTED_EDGE('',*,*,#15657,.T.);
#22452=ORIENTED_EDGE('',*,*,#15656,.T.);
#22453=ORIENTED_EDGE('',*,*,#15658,.F.);
#22454=ORIENTED_EDGE('',*,*,#15659,.F.);
#22455=ORIENTED_EDGE('',*,*,#15660,.T.);
#22456=ORIENTED_EDGE('',*,*,#15659,.T.);
#22457=ORIENTED_EDGE('',*,*,#15661,.F.);
#22458=ORIENTED_EDGE('',*,*,#15662,.F.);
#22459=ORIENTED_EDGE('',*,*,#15663,.T.);
#22460=ORIENTED_EDGE('',*,*,#15662,.T.);
#22461=ORIENTED_EDGE('',*,*,#15664,.F.);
#22462=ORIENTED_EDGE('',*,*,#15577,.F.);
#22463=ORIENTED_EDGE('',*,*,#15664,.T.);
#22464=ORIENTED_EDGE('',*,*,#15661,.T.);
#22465=ORIENTED_EDGE('',*,*,#15658,.T.);
#22466=ORIENTED_EDGE('',*,*,#15655,.T.);
#22467=ORIENTED_EDGE('',*,*,#15652,.T.);
#22468=ORIENTED_EDGE('',*,*,#15649,.T.);
#22469=ORIENTED_EDGE('',*,*,#15646,.T.);
#22470=ORIENTED_EDGE('',*,*,#15643,.T.);
#22471=ORIENTED_EDGE('',*,*,#15640,.T.);
#22472=ORIENTED_EDGE('',*,*,#15637,.T.);
#22473=ORIENTED_EDGE('',*,*,#15634,.T.);
#22474=ORIENTED_EDGE('',*,*,#15631,.T.);
#22475=ORIENTED_EDGE('',*,*,#15628,.T.);
#22476=ORIENTED_EDGE('',*,*,#15625,.T.);
#22477=ORIENTED_EDGE('',*,*,#15622,.T.);
#22478=ORIENTED_EDGE('',*,*,#15619,.T.);
#22479=ORIENTED_EDGE('',*,*,#15616,.T.);
#22480=ORIENTED_EDGE('',*,*,#15613,.T.);
#22481=ORIENTED_EDGE('',*,*,#15610,.T.);
#22482=ORIENTED_EDGE('',*,*,#15437,.T.);
#22483=ORIENTED_EDGE('',*,*,#15442,.T.);
#22484=ORIENTED_EDGE('',*,*,#15446,.T.);
#22485=ORIENTED_EDGE('',*,*,#15450,.T.);
#22486=ORIENTED_EDGE('',*,*,#15454,.T.);
#22487=ORIENTED_EDGE('',*,*,#15458,.T.);
#22488=ORIENTED_EDGE('',*,*,#15462,.T.);
#22489=ORIENTED_EDGE('',*,*,#15466,.T.);
#22490=ORIENTED_EDGE('',*,*,#15470,.T.);
#22491=ORIENTED_EDGE('',*,*,#15474,.T.);
#22492=ORIENTED_EDGE('',*,*,#15478,.T.);
#22493=ORIENTED_EDGE('',*,*,#15482,.T.);
#22494=ORIENTED_EDGE('',*,*,#15587,.T.);
#22495=ORIENTED_EDGE('',*,*,#15583,.T.);
#22496=ORIENTED_EDGE('',*,*,#15580,.T.);
#22497=ORIENTED_EDGE('',*,*,#15188,.T.);
#22498=ORIENTED_EDGE('',*,*,#15500,.F.);
#22499=ORIENTED_EDGE('',*,*,#15503,.F.);
#22500=ORIENTED_EDGE('',*,*,#15506,.F.);
#22501=ORIENTED_EDGE('',*,*,#15508,.F.);
#22502=ORIENTED_EDGE('',*,*,#15431,.F.);
#22503=ORIENTED_EDGE('',*,*,#15426,.F.);
#22504=ORIENTED_EDGE('',*,*,#15421,.F.);
#22505=ORIENTED_EDGE('',*,*,#15416,.F.);
#22506=ORIENTED_EDGE('',*,*,#15411,.F.);
#22507=ORIENTED_EDGE('',*,*,#15406,.F.);
#22508=ORIENTED_EDGE('',*,*,#15401,.F.);
#22509=ORIENTED_EDGE('',*,*,#15396,.F.);
#22510=ORIENTED_EDGE('',*,*,#15391,.F.);
#22511=ORIENTED_EDGE('',*,*,#15386,.F.);
#22512=ORIENTED_EDGE('',*,*,#15381,.F.);
#22513=ORIENTED_EDGE('',*,*,#15375,.F.);
#22514=ORIENTED_EDGE('',*,*,#15522,.F.);
#22515=ORIENTED_EDGE('',*,*,#15525,.F.);
#22516=ORIENTED_EDGE('',*,*,#15528,.F.);
#22517=ORIENTED_EDGE('',*,*,#15531,.F.);
#22518=ORIENTED_EDGE('',*,*,#15534,.F.);
#22519=ORIENTED_EDGE('',*,*,#15537,.F.);
#22520=ORIENTED_EDGE('',*,*,#15540,.F.);
#22521=ORIENTED_EDGE('',*,*,#15543,.F.);
#22522=ORIENTED_EDGE('',*,*,#15546,.F.);
#22523=ORIENTED_EDGE('',*,*,#15549,.F.);
#22524=ORIENTED_EDGE('',*,*,#15552,.F.);
#22525=ORIENTED_EDGE('',*,*,#15555,.F.);
#22526=ORIENTED_EDGE('',*,*,#15558,.F.);
#22527=ORIENTED_EDGE('',*,*,#15561,.F.);
#22528=ORIENTED_EDGE('',*,*,#15564,.F.);
#22529=ORIENTED_EDGE('',*,*,#15567,.F.);
#22530=ORIENTED_EDGE('',*,*,#15570,.F.);
#22531=ORIENTED_EDGE('',*,*,#15573,.F.);
#22532=ORIENTED_EDGE('',*,*,#15575,.F.);
#22533=ORIENTED_EDGE('',*,*,#15496,.F.);
#22534=ORIENTED_EDGE('',*,*,#15578,.T.);
#22535=ORIENTED_EDGE('',*,*,#15663,.F.);
#22536=ORIENTED_EDGE('',*,*,#15576,.T.);
#22537=ORIENTED_EDGE('',*,*,#15494,.F.);
#22538=ORIENTED_EDGE('',*,*,#15574,.T.);
#22539=ORIENTED_EDGE('',*,*,#15571,.T.);
#22540=ORIENTED_EDGE('',*,*,#15568,.T.);
#22541=ORIENTED_EDGE('',*,*,#15565,.F.);
#22542=ORIENTED_EDGE('',*,*,#15562,.T.);
#22543=ORIENTED_EDGE('',*,*,#15559,.T.);
#22544=ORIENTED_EDGE('',*,*,#15556,.T.);
#22545=ORIENTED_EDGE('',*,*,#15553,.T.);
#22546=ORIENTED_EDGE('',*,*,#15550,.T.);
#22547=ORIENTED_EDGE('',*,*,#15547,.T.);
#22548=ORIENTED_EDGE('',*,*,#15544,.T.);
#22549=ORIENTED_EDGE('',*,*,#15541,.T.);
#22550=ORIENTED_EDGE('',*,*,#15538,.T.);
#22551=ORIENTED_EDGE('',*,*,#15535,.F.);
#22552=ORIENTED_EDGE('',*,*,#15532,.T.);
#22553=ORIENTED_EDGE('',*,*,#15529,.T.);
#22554=ORIENTED_EDGE('',*,*,#15526,.T.);
#22555=ORIENTED_EDGE('',*,*,#15523,.T.);
#22556=ORIENTED_EDGE('',*,*,#15520,.T.);
#22557=ORIENTED_EDGE('',*,*,#15373,.T.);
#22558=ORIENTED_EDGE('',*,*,#15380,.T.);
#22559=ORIENTED_EDGE('',*,*,#15385,.F.);
#22560=ORIENTED_EDGE('',*,*,#15390,.T.);
#22561=ORIENTED_EDGE('',*,*,#15395,.F.);
#22562=ORIENTED_EDGE('',*,*,#15400,.T.);
#22563=ORIENTED_EDGE('',*,*,#15405,.F.);
#22564=ORIENTED_EDGE('',*,*,#15410,.T.);
#22565=ORIENTED_EDGE('',*,*,#15415,.F.);
#22566=ORIENTED_EDGE('',*,*,#15420,.T.);
#22567=ORIENTED_EDGE('',*,*,#15425,.F.);
#22568=ORIENTED_EDGE('',*,*,#15430,.T.);
#22569=ORIENTED_EDGE('',*,*,#15509,.T.);
#22570=ORIENTED_EDGE('',*,*,#15504,.T.);
#22571=ORIENTED_EDGE('',*,*,#15501,.T.);
#22572=ORIENTED_EDGE('',*,*,#15498,.T.);
#22573=ORIENTED_EDGE('',*,*,#15190,.F.);
#22574=ORIENTED_EDGE('',*,*,#15579,.F.);
#22575=ORIENTED_EDGE('',*,*,#15582,.F.);
#22576=ORIENTED_EDGE('',*,*,#15586,.F.);
#22577=ORIENTED_EDGE('',*,*,#15589,.F.);
#22578=ORIENTED_EDGE('',*,*,#15591,.T.);
#22579=ORIENTED_EDGE('',*,*,#15593,.F.);
#22580=ORIENTED_EDGE('',*,*,#15595,.T.);
#22581=ORIENTED_EDGE('',*,*,#15597,.F.);
#22582=ORIENTED_EDGE('',*,*,#15599,.T.);
#22583=ORIENTED_EDGE('',*,*,#15601,.F.);
#22584=ORIENTED_EDGE('',*,*,#15603,.T.);
#22585=ORIENTED_EDGE('',*,*,#15605,.F.);
#22586=ORIENTED_EDGE('',*,*,#15607,.T.);
#22587=ORIENTED_EDGE('',*,*,#15608,.F.);
#22588=ORIENTED_EDGE('',*,*,#15439,.F.);
#22589=ORIENTED_EDGE('',*,*,#15609,.F.);
#22590=ORIENTED_EDGE('',*,*,#15612,.F.);
#22591=ORIENTED_EDGE('',*,*,#15615,.F.);
#22592=ORIENTED_EDGE('',*,*,#15618,.F.);
#22593=ORIENTED_EDGE('',*,*,#15621,.F.);
#22594=ORIENTED_EDGE('',*,*,#15624,.T.);
#22595=ORIENTED_EDGE('',*,*,#15627,.F.);
#22596=ORIENTED_EDGE('',*,*,#15630,.F.);
#22597=ORIENTED_EDGE('',*,*,#15633,.F.);
#22598=ORIENTED_EDGE('',*,*,#15636,.F.);
#22599=ORIENTED_EDGE('',*,*,#15639,.F.);
#22600=ORIENTED_EDGE('',*,*,#15642,.F.);
#22601=ORIENTED_EDGE('',*,*,#15645,.F.);
#22602=ORIENTED_EDGE('',*,*,#15648,.F.);
#22603=ORIENTED_EDGE('',*,*,#15651,.F.);
#22604=ORIENTED_EDGE('',*,*,#15654,.T.);
#22605=ORIENTED_EDGE('',*,*,#15657,.F.);
#22606=ORIENTED_EDGE('',*,*,#15660,.F.);
#26501=PLANE('',#29156);
#26502=PLANE('',#29161);
#26503=PLANE('',#29162);
#26504=PLANE('',#29163);
#26505=PLANE('',#29183);
#26506=PLANE('',#29203);
#26507=PLANE('',#29226);
#26508=PLANE('',#29227);
#26509=PLANE('',#29228);
#26510=PLANE('',#29234);
#26511=PLANE('',#29235);
#26512=PLANE('',#29236);
#26513=PLANE('',#29242);
#26514=PLANE('',#29243);
#26515=PLANE('',#29244);
#26516=PLANE('',#29250);
#26517=PLANE('',#29251);
#26518=PLANE('',#29252);
#26519=PLANE('',#29258);
#26520=PLANE('',#29259);
#26521=PLANE('',#29260);
#26522=PLANE('',#29266);
#26523=PLANE('',#29267);
#26524=PLANE('',#29268);
#26525=PLANE('',#29272);
#26526=PLANE('',#29273);
#26527=PLANE('',#29274);
#26528=PLANE('',#29279);
#26529=PLANE('',#29280);
#26530=PLANE('',#29281);
#26531=PLANE('',#29286);
#26532=PLANE('',#29287);
#26533=PLANE('',#29288);
#26534=PLANE('',#29293);
#26535=PLANE('',#29294);
#26536=PLANE('',#29295);
#26537=PLANE('',#29300);
#26538=PLANE('',#29301);
#26539=PLANE('',#29302);
#26540=PLANE('',#29307);
#26541=PLANE('',#29308);
#26542=PLANE('',#29309);
#26543=PLANE('',#29319);
#26544=PLANE('',#29320);
#26545=PLANE('',#29324);
#26546=PLANE('',#29328);
#26547=PLANE('',#29330);
#26548=PLANE('',#29332);
#26549=PLANE('',#29334);
#26550=PLANE('',#29336);
#26551=PLANE('',#29338);
#26552=PLANE('',#29339);
#26553=PLANE('',#29343);
#26554=PLANE('',#29347);
#26555=PLANE('',#29351);
#26556=PLANE('',#29355);
#26557=PLANE('',#29359);
#26558=PLANE('',#29363);
#26559=PLANE('',#29364);
#26560=PLANE('',#29365);
#26561=PLANE('',#29369);
#26562=PLANE('',#29370);
#26563=PLANE('',#29371);
#26564=PLANE('',#29372);
#26565=PLANE('',#29376);
#26566=PLANE('',#29380);
#26567=PLANE('',#29383);
#26568=PLANE('',#29386);
#26569=PLANE('',#29389);
#26570=PLANE('',#29392);
#26571=PLANE('',#29395);
#26572=PLANE('',#29396);
#26573=PLANE('',#29400);
#26574=PLANE('',#29404);
#26575=PLANE('',#29408);
#26576=PLANE('',#29412);
#26577=PLANE('',#29416);
#26578=PLANE('',#29420);
#26579=PLANE('',#29421);
#26580=PLANE('',#29422);
#26581=PLANE('',#29426);
#26582=PLANE('',#29427);
#26583=PLANE('',#29428);
#26584=PLANE('',#29429);
#26585=PLANE('',#29430);
#27402=ADVANCED_FACE('',(#3599),#2564,.F.);
#27403=ADVANCED_FACE('',(#3600),#26501,.T.);
#27404=ADVANCED_FACE('',(#3601),#2565,.F.);
#27405=ADVANCED_FACE('',(#3602),#26502,.T.);
#27406=ADVANCED_FACE('',(#3603),#26503,.T.);
#27407=ADVANCED_FACE('',(#3604),#26504,.T.);
#27408=ADVANCED_FACE('',(#3605),#2566,.F.);
#27409=ADVANCED_FACE('',(#3606),#26505,.T.);
#27410=ADVANCED_FACE('',(#3607),#2567,.F.);
#27411=ADVANCED_FACE('',(#3608),#26506,.T.);
#27412=ADVANCED_FACE('',(#3609),#2568,.F.);
#27413=ADVANCED_FACE('',(#3610),#2569,.T.);
#27414=ADVANCED_FACE('',(#3611),#26507,.F.);
#27415=ADVANCED_FACE('',(#3612),#26508,.F.);
#27416=ADVANCED_FACE('',(#3613),#26509,.F.);
#27417=ADVANCED_FACE('',(#3614),#2570,.F.);
#27418=ADVANCED_FACE('',(#3615),#2571,.F.);
#27419=ADVANCED_FACE('',(#3616),#2572,.F.);
#27420=ADVANCED_FACE('',(#3617),#26510,.F.);
#27421=ADVANCED_FACE('',(#3618),#26511,.F.);
#27422=ADVANCED_FACE('',(#3619),#26512,.F.);
#27423=ADVANCED_FACE('',(#3620),#2573,.F.);
#27424=ADVANCED_FACE('',(#3621),#2574,.F.);
#27425=ADVANCED_FACE('',(#3622),#2575,.F.);
#27426=ADVANCED_FACE('',(#3623),#26513,.F.);
#27427=ADVANCED_FACE('',(#3624),#26514,.F.);
#27428=ADVANCED_FACE('',(#3625),#26515,.F.);
#27429=ADVANCED_FACE('',(#3626),#2576,.F.);
#27430=ADVANCED_FACE('',(#3627),#2577,.F.);
#27431=ADVANCED_FACE('',(#3628),#2578,.F.);
#27432=ADVANCED_FACE('',(#3629),#26516,.F.);
#27433=ADVANCED_FACE('',(#3630),#26517,.F.);
#27434=ADVANCED_FACE('',(#3631),#26518,.F.);
#27435=ADVANCED_FACE('',(#3632),#2579,.F.);
#27436=ADVANCED_FACE('',(#3633),#2580,.F.);
#27437=ADVANCED_FACE('',(#3634),#2581,.F.);
#27438=ADVANCED_FACE('',(#3635),#26519,.F.);
#27439=ADVANCED_FACE('',(#3636),#26520,.F.);
#27440=ADVANCED_FACE('',(#3637),#26521,.F.);
#27441=ADVANCED_FACE('',(#3638),#2582,.F.);
#27442=ADVANCED_FACE('',(#3639),#2583,.F.);
#27443=ADVANCED_FACE('',(#3640),#2584,.F.);
#27444=ADVANCED_FACE('',(#3641),#26522,.F.);
#27445=ADVANCED_FACE('',(#3642),#26523,.F.);
#27446=ADVANCED_FACE('',(#3643),#26524,.F.);
#27447=ADVANCED_FACE('',(#3644),#2585,.T.);
#27448=ADVANCED_FACE('',(#3645),#26525,.T.);
#27449=ADVANCED_FACE('',(#3646),#26526,.T.);
#27450=ADVANCED_FACE('',(#3647),#26527,.T.);
#27451=ADVANCED_FACE('',(#3648),#2586,.F.);
#27452=ADVANCED_FACE('',(#3649),#2587,.F.);
#27453=ADVANCED_FACE('',(#3650),#2588,.F.);
#27454=ADVANCED_FACE('',(#3651),#26528,.T.);
#27455=ADVANCED_FACE('',(#3652),#26529,.T.);
#27456=ADVANCED_FACE('',(#3653),#26530,.T.);
#27457=ADVANCED_FACE('',(#3654),#2589,.F.);
#27458=ADVANCED_FACE('',(#3655),#2590,.F.);
#27459=ADVANCED_FACE('',(#3656),#2591,.F.);
#27460=ADVANCED_FACE('',(#3657),#26531,.T.);
#27461=ADVANCED_FACE('',(#3658),#26532,.T.);
#27462=ADVANCED_FACE('',(#3659),#26533,.T.);
#27463=ADVANCED_FACE('',(#3660),#2592,.F.);
#27464=ADVANCED_FACE('',(#3661),#2593,.F.);
#27465=ADVANCED_FACE('',(#3662),#2594,.F.);
#27466=ADVANCED_FACE('',(#3663),#26534,.T.);
#27467=ADVANCED_FACE('',(#3664),#26535,.T.);
#27468=ADVANCED_FACE('',(#3665),#26536,.T.);
#27469=ADVANCED_FACE('',(#3666),#2595,.F.);
#27470=ADVANCED_FACE('',(#3667),#2596,.F.);
#27471=ADVANCED_FACE('',(#3668),#2597,.F.);
#27472=ADVANCED_FACE('',(#3669),#26537,.T.);
#27473=ADVANCED_FACE('',(#3670),#26538,.T.);
#27474=ADVANCED_FACE('',(#3671),#26539,.T.);
#27475=ADVANCED_FACE('',(#3672),#2598,.F.);
#27476=ADVANCED_FACE('',(#3673),#2599,.F.);
#27477=ADVANCED_FACE('',(#3674),#2600,.F.);
#27478=ADVANCED_FACE('',(#3675),#26540,.T.);
#27479=ADVANCED_FACE('',(#3676),#26541,.T.);
#27480=ADVANCED_FACE('',(#3677),#26542,.T.);
#27481=ADVANCED_FACE('',(#3678),#2601,.F.);
#27482=ADVANCED_FACE('',(#3679),#2602,.F.);
#27483=ADVANCED_FACE('',(#3680),#2603,.F.);
#27484=ADVANCED_FACE('',(#3681),#26543,.F.);
#27485=ADVANCED_FACE('',(#3682),#26544,.F.);
#27486=ADVANCED_FACE('',(#3683),#2604,.T.);
#27487=ADVANCED_FACE('',(#3684),#26545,.F.);
#27488=ADVANCED_FACE('',(#3685),#2605,.T.);
#27489=ADVANCED_FACE('',(#3686),#26546,.F.);
#27490=ADVANCED_FACE('',(#3687),#2606,.F.);
#27491=ADVANCED_FACE('',(#3688),#26547,.F.);
#27492=ADVANCED_FACE('',(#3689),#2607,.F.);
#27493=ADVANCED_FACE('',(#3690),#26548,.F.);
#27494=ADVANCED_FACE('',(#3691),#2608,.F.);
#27495=ADVANCED_FACE('',(#3692),#26549,.F.);
#27496=ADVANCED_FACE('',(#3693),#2609,.F.);
#27497=ADVANCED_FACE('',(#3694),#26550,.F.);
#27498=ADVANCED_FACE('',(#3695),#2610,.F.);
#27499=ADVANCED_FACE('',(#3696),#26551,.F.);
#27500=ADVANCED_FACE('',(#3697),#26552,.F.);
#27501=ADVANCED_FACE('',(#3698),#2611,.T.);
#27502=ADVANCED_FACE('',(#3699),#26553,.F.);
#27503=ADVANCED_FACE('',(#3700),#2612,.T.);
#27504=ADVANCED_FACE('',(#3701,#204,#205,#206),#26554,.F.);
#27505=ADVANCED_FACE('',(#3702),#2613,.F.);
#27506=ADVANCED_FACE('',(#3703),#26555,.F.);
#27507=ADVANCED_FACE('',(#3704),#2614,.T.);
#27508=ADVANCED_FACE('',(#3705),#26556,.F.);
#27509=ADVANCED_FACE('',(#3706),#2615,.T.);
#27510=ADVANCED_FACE('',(#3707,#207,#208,#209),#26557,.F.);
#27511=ADVANCED_FACE('',(#3708),#2616,.T.);
#27512=ADVANCED_FACE('',(#3709),#26558,.F.);
#27513=ADVANCED_FACE('',(#3710),#26559,.F.);
#27514=ADVANCED_FACE('',(#3711,#210,#211,#212),#26560,.F.);
#27515=ADVANCED_FACE('',(#3712),#2617,.F.);
#27516=ADVANCED_FACE('',(#3713),#26561,.F.);
#27517=ADVANCED_FACE('',(#3714),#26562,.F.);
#27518=ADVANCED_FACE('',(#3715),#26563,.F.);
#27519=ADVANCED_FACE('',(#3716),#26564,.T.);
#27520=ADVANCED_FACE('',(#3717),#2618,.T.);
#27521=ADVANCED_FACE('',(#3718),#26565,.T.);
#27522=ADVANCED_FACE('',(#3719),#2619,.T.);
#27523=ADVANCED_FACE('',(#3720),#26566,.T.);
#27524=ADVANCED_FACE('',(#3721),#2620,.F.);
#27525=ADVANCED_FACE('',(#3722),#26567,.T.);
#27526=ADVANCED_FACE('',(#3723),#2621,.F.);
#27527=ADVANCED_FACE('',(#3724),#26568,.T.);
#27528=ADVANCED_FACE('',(#3725),#2622,.F.);
#27529=ADVANCED_FACE('',(#3726),#26569,.T.);
#27530=ADVANCED_FACE('',(#3727),#2623,.F.);
#27531=ADVANCED_FACE('',(#3728),#26570,.T.);
#27532=ADVANCED_FACE('',(#3729),#2624,.F.);
#27533=ADVANCED_FACE('',(#3730),#26571,.T.);
#27534=ADVANCED_FACE('',(#3731),#26572,.T.);
#27535=ADVANCED_FACE('',(#3732),#2625,.T.);
#27536=ADVANCED_FACE('',(#3733),#26573,.T.);
#27537=ADVANCED_FACE('',(#3734),#2626,.T.);
#27538=ADVANCED_FACE('',(#3735,#213,#214,#215),#26574,.T.);
#27539=ADVANCED_FACE('',(#3736),#2627,.F.);
#27540=ADVANCED_FACE('',(#3737),#26575,.T.);
#27541=ADVANCED_FACE('',(#3738),#2628,.T.);
#27542=ADVANCED_FACE('',(#3739),#26576,.T.);
#27543=ADVANCED_FACE('',(#3740),#2629,.T.);
#27544=ADVANCED_FACE('',(#3741),#26577,.T.);
#27545=ADVANCED_FACE('',(#3742),#2630,.T.);
#27546=ADVANCED_FACE('',(#3743),#26578,.T.);
#27547=ADVANCED_FACE('',(#3744),#26579,.T.);
#27548=ADVANCED_FACE('',(#3745),#26580,.T.);
#27549=ADVANCED_FACE('',(#3746),#2631,.F.);
#27550=ADVANCED_FACE('',(#3747),#26581,.T.);
#27551=ADVANCED_FACE('',(#3748),#26582,.T.);
#27552=ADVANCED_FACE('',(#3749),#26583,.T.);
#27553=ADVANCED_FACE('',(#3750),#26584,.T.);
#27554=ADVANCED_FACE('',(#3751),#26585,.F.);
#28085=CLOSED_SHELL('',(#27402,#27403,#27404,#27405,#27406,#27407,#27408,
#27409,#27410,#27411,#27412,#27413,#27414,#27415,#27416,#27417,#27418,#27419,
#27420,#27421,#27422,#27423,#27424,#27425,#27426,#27427,#27428,#27429,#27430,
#27431,#27432,#27433,#27434,#27435,#27436,#27437,#27438,#27439,#27440,#27441,
#27442,#27443,#27444,#27445,#27446,#27447,#27448,#27449,#27450,#27451,#27452,
#27453,#27454,#27455,#27456,#27457,#27458,#27459,#27460,#27461,#27462,#27463,
#27464,#27465,#27466,#27467,#27468,#27469,#27470,#27471,#27472,#27473,#27474,
#27475,#27476,#27477,#27478,#27479,#27480,#27481,#27482,#27483,#27484,#27485,
#27486,#27487,#27488,#27489,#27490,#27491,#27492,#27493,#27494,#27495,#27496,
#27497,#27498,#27499,#27500,#27501,#27502,#27503,#27504,#27505,#27506,#27507,
#27508,#27509,#27510,#27511,#27512,#27513,#27514,#27515,#27516,#27517,#27518,
#27519,#27520,#27521,#27522,#27523,#27524,#27525,#27526,#27527,#27528,#27529,
#27530,#27531,#27532,#27533,#27534,#27535,#27536,#27537,#27538,#27539,#27540,
#27541,#27542,#27543,#27544,#27545,#27546,#27547,#27548,#27549,#27550,#27551,
#27552,#27553,#27554));
#28709=AXIS2_PLACEMENT_3D('',#124427,#31762,#31763);
#29152=AXIS2_PLACEMENT_3D('',#125618,#32904,#32905);
#29153=AXIS2_PLACEMENT_3D('',#125621,#32906,#32907);
#29154=AXIS2_PLACEMENT_3D('',#125622,#32908,#32909);
#29155=AXIS2_PLACEMENT_3D('',#125625,#32911,#32912);
#29156=AXIS2_PLACEMENT_3D('',#125626,#32913,#32914);
#29157=AXIS2_PLACEMENT_3D('',#125627,#32915,#32916);
#29158=AXIS2_PLACEMENT_3D('',#125630,#32917,#32918);
#29159=AXIS2_PLACEMENT_3D('',#125631,#32919,#32920);
#29160=AXIS2_PLACEMENT_3D('',#125634,#32922,#32923);
#29161=AXIS2_PLACEMENT_3D('',#125635,#32924,#32925);
#29162=AXIS2_PLACEMENT_3D('',#125636,#32926,#32927);
#29163=AXIS2_PLACEMENT_3D('',#125647,#32934,#32935);
#29164=AXIS2_PLACEMENT_3D('',#125651,#32937,#32938);
#29165=AXIS2_PLACEMENT_3D('',#125652,#32939,#32940);
#29166=AXIS2_PLACEMENT_3D('',#125654,#32941,#32942);
#29167=AXIS2_PLACEMENT_3D('',#125663,#32944,#32945);
#29168=AXIS2_PLACEMENT_3D('',#125718,#32948,#32949);
#29169=AXIS2_PLACEMENT_3D('',#125727,#32950,#32951);
#29170=AXIS2_PLACEMENT_3D('',#125745,#32953,#32954);
#29171=AXIS2_PLACEMENT_3D('',#125812,#32957,#32958);
#29172=AXIS2_PLACEMENT_3D('',#125816,#32960,#32961);
#29173=AXIS2_PLACEMENT_3D('',#125883,#32964,#32965);
#29174=AXIS2_PLACEMENT_3D('',#125903,#32967,#32968);
#29175=AXIS2_PLACEMENT_3D('',#125916,#32969,#32970);
#29176=AXIS2_PLACEMENT_3D('',#125984,#32973,#32974);
#29177=AXIS2_PLACEMENT_3D('',#125994,#32976,#32977);
#29178=AXIS2_PLACEMENT_3D('',#125995,#32978,#32979);
#29179=AXIS2_PLACEMENT_3D('',#126006,#32980,#32981);
#29180=AXIS2_PLACEMENT_3D('',#126026,#32983,#32984);
#29181=AXIS2_PLACEMENT_3D('',#126028,#32985,#32986);
#29182=AXIS2_PLACEMENT_3D('',#126046,#32988,#32989);
#29183=AXIS2_PLACEMENT_3D('',#126053,#32990,#32991);
#29184=AXIS2_PLACEMENT_3D('',#126057,#32993,#32994);
#29185=AXIS2_PLACEMENT_3D('',#126058,#32995,#32996);
#29186=AXIS2_PLACEMENT_3D('',#126060,#32997,#32998);
#29187=AXIS2_PLACEMENT_3D('',#126069,#33000,#33001);
#29188=AXIS2_PLACEMENT_3D('',#126124,#33004,#33005);
#29189=AXIS2_PLACEMENT_3D('',#126133,#33006,#33007);
#29190=AXIS2_PLACEMENT_3D('',#126151,#33009,#33010);
#29191=AXIS2_PLACEMENT_3D('',#126218,#33013,#33014);
#29192=AXIS2_PLACEMENT_3D('',#126222,#33016,#33017);
#29193=AXIS2_PLACEMENT_3D('',#126289,#33020,#33021);
#29194=AXIS2_PLACEMENT_3D('',#126309,#33023,#33024);
#29195=AXIS2_PLACEMENT_3D('',#126322,#33025,#33026);
#29196=AXIS2_PLACEMENT_3D('',#126390,#33029,#33030);
#29197=AXIS2_PLACEMENT_3D('',#126400,#33032,#33033);
#29198=AXIS2_PLACEMENT_3D('',#126401,#33034,#33035);
#29199=AXIS2_PLACEMENT_3D('',#126412,#33036,#33037);
#29200=AXIS2_PLACEMENT_3D('',#126432,#33039,#33040);
#29201=AXIS2_PLACEMENT_3D('',#126434,#33041,#33042);
#29202=AXIS2_PLACEMENT_3D('',#126452,#33044,#33045);
#29203=AXIS2_PLACEMENT_3D('',#126459,#33046,#33047);
#29204=AXIS2_PLACEMENT_3D('',#126463,#33049,#33050);
#29205=AXIS2_PLACEMENT_3D('',#126464,#33051,#33052);
#29206=AXIS2_PLACEMENT_3D('',#126466,#33053,#33054);
#29207=AXIS2_PLACEMENT_3D('',#126475,#33056,#33057);
#29208=AXIS2_PLACEMENT_3D('',#126534,#33060,#33061);
#29209=AXIS2_PLACEMENT_3D('',#126543,#33062,#33063);
#29210=AXIS2_PLACEMENT_3D('',#126561,#33065,#33066);
#29211=AXIS2_PLACEMENT_3D('',#126628,#33069,#33070);
#29212=AXIS2_PLACEMENT_3D('',#126632,#33072,#33073);
#29213=AXIS2_PLACEMENT_3D('',#126699,#33076,#33077);
#29214=AXIS2_PLACEMENT_3D('',#126719,#33079,#33080);
#29215=AXIS2_PLACEMENT_3D('',#126732,#33081,#33082);
#29216=AXIS2_PLACEMENT_3D('',#126800,#33085,#33086);
#29217=AXIS2_PLACEMENT_3D('',#126810,#33088,#33089);
#29218=AXIS2_PLACEMENT_3D('',#126811,#33090,#33091);
#29219=AXIS2_PLACEMENT_3D('',#126822,#33092,#33093);
#29220=AXIS2_PLACEMENT_3D('',#126842,#33095,#33096);
#29221=AXIS2_PLACEMENT_3D('',#126844,#33097,#33098);
#29222=AXIS2_PLACEMENT_3D('',#126862,#33100,#33101);
#29223=AXIS2_PLACEMENT_3D('',#126869,#33102,#33103);
#29224=AXIS2_PLACEMENT_3D('',#126873,#33105,#33106);
#29225=AXIS2_PLACEMENT_3D('',#126877,#33108,#33109);
#29226=AXIS2_PLACEMENT_3D('',#126881,#33113,#33114);
#29227=AXIS2_PLACEMENT_3D('',#126885,#33117,#33118);
#29228=AXIS2_PLACEMENT_3D('',#126889,#33121,#33122);
#29229=AXIS2_PLACEMENT_3D('',#126891,#33124,#33125);
#29230=AXIS2_PLACEMENT_3D('',#126894,#33127,#33128);
#29231=AXIS2_PLACEMENT_3D('',#126895,#33129,#33130);
#29232=AXIS2_PLACEMENT_3D('',#126897,#33131,#33132);
#29233=AXIS2_PLACEMENT_3D('',#126899,#33134,#33135);
#29234=AXIS2_PLACEMENT_3D('',#126901,#33137,#33138);
#29235=AXIS2_PLACEMENT_3D('',#126905,#33141,#33142);
#29236=AXIS2_PLACEMENT_3D('',#126909,#33145,#33146);
#29237=AXIS2_PLACEMENT_3D('',#126911,#33148,#33149);
#29238=AXIS2_PLACEMENT_3D('',#126914,#33151,#33152);
#29239=AXIS2_PLACEMENT_3D('',#126915,#33153,#33154);
#29240=AXIS2_PLACEMENT_3D('',#126917,#33155,#33156);
#29241=AXIS2_PLACEMENT_3D('',#126919,#33158,#33159);
#29242=AXIS2_PLACEMENT_3D('',#126921,#33161,#33162);
#29243=AXIS2_PLACEMENT_3D('',#126925,#33165,#33166);
#29244=AXIS2_PLACEMENT_3D('',#126929,#33169,#33170);
#29245=AXIS2_PLACEMENT_3D('',#126931,#33172,#33173);
#29246=AXIS2_PLACEMENT_3D('',#126934,#33175,#33176);
#29247=AXIS2_PLACEMENT_3D('',#126935,#33177,#33178);
#29248=AXIS2_PLACEMENT_3D('',#126937,#33179,#33180);
#29249=AXIS2_PLACEMENT_3D('',#126939,#33182,#33183);
#29250=AXIS2_PLACEMENT_3D('',#126941,#33185,#33186);
#29251=AXIS2_PLACEMENT_3D('',#126945,#33189,#33190);
#29252=AXIS2_PLACEMENT_3D('',#126949,#33193,#33194);
#29253=AXIS2_PLACEMENT_3D('',#126951,#33196,#33197);
#29254=AXIS2_PLACEMENT_3D('',#126954,#33199,#33200);
#29255=AXIS2_PLACEMENT_3D('',#126955,#33201,#33202);
#29256=AXIS2_PLACEMENT_3D('',#126957,#33203,#33204);
#29257=AXIS2_PLACEMENT_3D('',#126959,#33206,#33207);
#29258=AXIS2_PLACEMENT_3D('',#126961,#33209,#33210);
#29259=AXIS2_PLACEMENT_3D('',#126965,#33213,#33214);
#29260=AXIS2_PLACEMENT_3D('',#126969,#33217,#33218);
#29261=AXIS2_PLACEMENT_3D('',#126971,#33220,#33221);
#29262=AXIS2_PLACEMENT_3D('',#126974,#33223,#33224);
#29263=AXIS2_PLACEMENT_3D('',#126975,#33225,#33226);
#29264=AXIS2_PLACEMENT_3D('',#126977,#33227,#33228);
#29265=AXIS2_PLACEMENT_3D('',#126979,#33230,#33231);
#29266=AXIS2_PLACEMENT_3D('',#126981,#33233,#33234);
#29267=AXIS2_PLACEMENT_3D('',#126985,#33237,#33238);
#29268=AXIS2_PLACEMENT_3D('',#126989,#33241,#33242);
#29269=AXIS2_PLACEMENT_3D('',#126991,#33244,#33245);
#29270=AXIS2_PLACEMENT_3D('',#126997,#33249,#33250);
#29271=AXIS2_PLACEMENT_3D('',#127001,#33252,#33253);
#29272=AXIS2_PLACEMENT_3D('',#127003,#33255,#33256);
#29273=AXIS2_PLACEMENT_3D('',#127007,#33259,#33260);
#29274=AXIS2_PLACEMENT_3D('',#127009,#33262,#33263);
#29275=AXIS2_PLACEMENT_3D('',#127011,#33265,#33266);
#29276=AXIS2_PLACEMENT_3D('',#127014,#33268,#33269);
#29277=AXIS2_PLACEMENT_3D('',#127015,#33270,#33271);
#29278=AXIS2_PLACEMENT_3D('',#127017,#33273,#33274);
#29279=AXIS2_PLACEMENT_3D('',#127019,#33276,#33277);
#29280=AXIS2_PLACEMENT_3D('',#127023,#33280,#33281);
#29281=AXIS2_PLACEMENT_3D('',#127025,#33283,#33284);
#29282=AXIS2_PLACEMENT_3D('',#127027,#33286,#33287);
#29283=AXIS2_PLACEMENT_3D('',#127030,#33289,#33290);
#29284=AXIS2_PLACEMENT_3D('',#127031,#33291,#33292);
#29285=AXIS2_PLACEMENT_3D('',#127033,#33294,#33295);
#29286=AXIS2_PLACEMENT_3D('',#127035,#33297,#33298);
#29287=AXIS2_PLACEMENT_3D('',#127039,#33301,#33302);
#29288=AXIS2_PLACEMENT_3D('',#127041,#33304,#33305);
#29289=AXIS2_PLACEMENT_3D('',#127043,#33307,#33308);
#29290=AXIS2_PLACEMENT_3D('',#127046,#33310,#33311);
#29291=AXIS2_PLACEMENT_3D('',#127047,#33312,#33313);
#29292=AXIS2_PLACEMENT_3D('',#127049,#33315,#33316);
#29293=AXIS2_PLACEMENT_3D('',#127051,#33318,#33319);
#29294=AXIS2_PLACEMENT_3D('',#127055,#33322,#33323);
#29295=AXIS2_PLACEMENT_3D('',#127057,#33325,#33326);
#29296=AXIS2_PLACEMENT_3D('',#127059,#33328,#33329);
#29297=AXIS2_PLACEMENT_3D('',#127062,#33331,#33332);
#29298=AXIS2_PLACEMENT_3D('',#127063,#33333,#33334);
#29299=AXIS2_PLACEMENT_3D('',#127065,#33336,#33337);
#29300=AXIS2_PLACEMENT_3D('',#127067,#33339,#33340);
#29301=AXIS2_PLACEMENT_3D('',#127071,#33343,#33344);
#29302=AXIS2_PLACEMENT_3D('',#127073,#33346,#33347);
#29303=AXIS2_PLACEMENT_3D('',#127075,#33349,#33350);
#29304=AXIS2_PLACEMENT_3D('',#127078,#33352,#33353);
#29305=AXIS2_PLACEMENT_3D('',#127079,#33354,#33355);
#29306=AXIS2_PLACEMENT_3D('',#127081,#33357,#33358);
#29307=AXIS2_PLACEMENT_3D('',#127083,#33360,#33361);
#29308=AXIS2_PLACEMENT_3D('',#127087,#33364,#33365);
#29309=AXIS2_PLACEMENT_3D('',#127089,#33367,#33368);
#29310=AXIS2_PLACEMENT_3D('',#127091,#33370,#33371);
#29311=AXIS2_PLACEMENT_3D('',#127093,#33372,#33373);
#29312=AXIS2_PLACEMENT_3D('',#127096,#33375,#33376);
#29313=AXIS2_PLACEMENT_3D('',#127097,#33377,#33378);
#29314=AXIS2_PLACEMENT_3D('',#127099,#33379,#33380);
#29315=AXIS2_PLACEMENT_3D('',#127102,#33382,#33383);
#29316=AXIS2_PLACEMENT_3D('',#127103,#33384,#33385);
#29317=AXIS2_PLACEMENT_3D('',#127105,#33386,#33387);
#29318=AXIS2_PLACEMENT_3D('',#127108,#33389,#33390);
#29319=AXIS2_PLACEMENT_3D('',#127109,#33391,#33392);
#29320=AXIS2_PLACEMENT_3D('',#127118,#33397,#33398);
#29321=AXIS2_PLACEMENT_3D('',#127124,#33402,#33403);
#29322=AXIS2_PLACEMENT_3D('',#127126,#33404,#33405);
#29323=AXIS2_PLACEMENT_3D('',#127129,#33407,#33408);
#29324=AXIS2_PLACEMENT_3D('',#127130,#33409,#33410);
#29325=AXIS2_PLACEMENT_3D('',#127136,#33414,#33415);
#29326=AXIS2_PLACEMENT_3D('',#127138,#33417,#33418);
#29327=AXIS2_PLACEMENT_3D('',#127139,#33419,#33420);
#29328=AXIS2_PLACEMENT_3D('',#127140,#33421,#33422);
#29329=AXIS2_PLACEMENT_3D('',#127142,#33424,#33425);
#29330=AXIS2_PLACEMENT_3D('',#127144,#33427,#33428);
#29331=AXIS2_PLACEMENT_3D('',#127146,#33430,#33431);
#29332=AXIS2_PLACEMENT_3D('',#127148,#33433,#33434);
#29333=AXIS2_PLACEMENT_3D('',#127150,#33436,#33437);
#29334=AXIS2_PLACEMENT_3D('',#127152,#33439,#33440);
#29335=AXIS2_PLACEMENT_3D('',#127154,#33442,#33443);
#29336=AXIS2_PLACEMENT_3D('',#127156,#33445,#33446);
#29337=AXIS2_PLACEMENT_3D('',#127158,#33448,#33449);
#29338=AXIS2_PLACEMENT_3D('',#127160,#33451,#33452);
#29339=AXIS2_PLACEMENT_3D('',#127161,#33453,#33454);
#29340=AXIS2_PLACEMENT_3D('',#127167,#33458,#33459);
#29341=AXIS2_PLACEMENT_3D('',#127169,#33460,#33461);
#29342=AXIS2_PLACEMENT_3D('',#127172,#33463,#33464);
#29343=AXIS2_PLACEMENT_3D('',#127173,#33465,#33466);
#29344=AXIS2_PLACEMENT_3D('',#127179,#33470,#33471);
#29345=AXIS2_PLACEMENT_3D('',#127181,#33472,#33473);
#29346=AXIS2_PLACEMENT_3D('',#127184,#33475,#33476);
#29347=AXIS2_PLACEMENT_3D('',#127185,#33477,#33478);
#29348=AXIS2_PLACEMENT_3D('',#127191,#33482,#33483);
#29349=AXIS2_PLACEMENT_3D('',#127193,#33484,#33485);
#29350=AXIS2_PLACEMENT_3D('',#127196,#33487,#33488);
#29351=AXIS2_PLACEMENT_3D('',#127197,#33489,#33490);
#29352=AXIS2_PLACEMENT_3D('',#127203,#33494,#33495);
#29353=AXIS2_PLACEMENT_3D('',#127205,#33496,#33497);
#29354=AXIS2_PLACEMENT_3D('',#127208,#33499,#33500);
#29355=AXIS2_PLACEMENT_3D('',#127209,#33501,#33502);
#29356=AXIS2_PLACEMENT_3D('',#127215,#33506,#33507);
#29357=AXIS2_PLACEMENT_3D('',#127217,#33508,#33509);
#29358=AXIS2_PLACEMENT_3D('',#127220,#33511,#33512);
#29359=AXIS2_PLACEMENT_3D('',#127221,#33513,#33514);
#29360=AXIS2_PLACEMENT_3D('',#127227,#33518,#33519);
#29361=AXIS2_PLACEMENT_3D('',#127229,#33520,#33521);
#29362=AXIS2_PLACEMENT_3D('',#127232,#33523,#33524);
#29363=AXIS2_PLACEMENT_3D('',#127233,#33525,#33526);
#29364=AXIS2_PLACEMENT_3D('',#127239,#33530,#33531);
#29365=AXIS2_PLACEMENT_3D('',#127245,#33535,#33536);
#29366=AXIS2_PLACEMENT_3D('',#127251,#33540,#33541);
#29367=AXIS2_PLACEMENT_3D('',#127253,#33542,#33543);
#29368=AXIS2_PLACEMENT_3D('',#127256,#33545,#33546);
#29369=AXIS2_PLACEMENT_3D('',#127257,#33547,#33548);
#29370=AXIS2_PLACEMENT_3D('',#127263,#33552,#33553);
#29371=AXIS2_PLACEMENT_3D('',#127269,#33557,#33558);
#29372=AXIS2_PLACEMENT_3D('',#127272,#33561,#33562);
#29373=AXIS2_PLACEMENT_3D('',#127278,#33566,#33567);
#29374=AXIS2_PLACEMENT_3D('',#127280,#33568,#33569);
#29375=AXIS2_PLACEMENT_3D('',#127282,#33570,#33571);
#29376=AXIS2_PLACEMENT_3D('',#127284,#33573,#33574);
#29377=AXIS2_PLACEMENT_3D('',#127290,#33578,#33579);
#29378=AXIS2_PLACEMENT_3D('',#127293,#33581,#33582);
#29379=AXIS2_PLACEMENT_3D('',#127294,#33583,#33584);
#29380=AXIS2_PLACEMENT_3D('',#127295,#33585,#33586);
#29381=AXIS2_PLACEMENT_3D('',#127299,#33589,#33590);
#29382=AXIS2_PLACEMENT_3D('',#127302,#33592,#33593);
#29383=AXIS2_PLACEMENT_3D('',#127303,#33594,#33595);
#29384=AXIS2_PLACEMENT_3D('',#127307,#33598,#33599);
#29385=AXIS2_PLACEMENT_3D('',#127310,#33601,#33602);
#29386=AXIS2_PLACEMENT_3D('',#127311,#33603,#33604);
#29387=AXIS2_PLACEMENT_3D('',#127315,#33607,#33608);
#29388=AXIS2_PLACEMENT_3D('',#127318,#33610,#33611);
#29389=AXIS2_PLACEMENT_3D('',#127319,#33612,#33613);
#29390=AXIS2_PLACEMENT_3D('',#127323,#33616,#33617);
#29391=AXIS2_PLACEMENT_3D('',#127326,#33619,#33620);
#29392=AXIS2_PLACEMENT_3D('',#127327,#33621,#33622);
#29393=AXIS2_PLACEMENT_3D('',#127331,#33625,#33626);
#29394=AXIS2_PLACEMENT_3D('',#127334,#33628,#33629);
#29395=AXIS2_PLACEMENT_3D('',#127335,#33630,#33631);
#29396=AXIS2_PLACEMENT_3D('',#127337,#33633,#33634);
#29397=AXIS2_PLACEMENT_3D('',#127343,#33638,#33639);
#29398=AXIS2_PLACEMENT_3D('',#127345,#33640,#33641);
#29399=AXIS2_PLACEMENT_3D('',#127347,#33642,#33643);
#29400=AXIS2_PLACEMENT_3D('',#127349,#33645,#33646);
#29401=AXIS2_PLACEMENT_3D('',#127355,#33650,#33651);
#29402=AXIS2_PLACEMENT_3D('',#127357,#33652,#33653);
#29403=AXIS2_PLACEMENT_3D('',#127359,#33654,#33655);
#29404=AXIS2_PLACEMENT_3D('',#127361,#33657,#33658);
#29405=AXIS2_PLACEMENT_3D('',#127367,#33662,#33663);
#29406=AXIS2_PLACEMENT_3D('',#127369,#33664,#33665);
#29407=AXIS2_PLACEMENT_3D('',#127371,#33666,#33667);
#29408=AXIS2_PLACEMENT_3D('',#127373,#33669,#33670);
#29409=AXIS2_PLACEMENT_3D('',#127379,#33674,#33675);
#29410=AXIS2_PLACEMENT_3D('',#127381,#33676,#33677);
#29411=AXIS2_PLACEMENT_3D('',#127383,#33678,#33679);
#29412=AXIS2_PLACEMENT_3D('',#127385,#33681,#33682);
#29413=AXIS2_PLACEMENT_3D('',#127391,#33686,#33687);
#29414=AXIS2_PLACEMENT_3D('',#127393,#33688,#33689);
#29415=AXIS2_PLACEMENT_3D('',#127395,#33690,#33691);
#29416=AXIS2_PLACEMENT_3D('',#127397,#33693,#33694);
#29417=AXIS2_PLACEMENT_3D('',#127403,#33698,#33699);
#29418=AXIS2_PLACEMENT_3D('',#127405,#33700,#33701);
#29419=AXIS2_PLACEMENT_3D('',#127407,#33702,#33703);
#29420=AXIS2_PLACEMENT_3D('',#127409,#33705,#33706);
#29421=AXIS2_PLACEMENT_3D('',#127415,#33710,#33711);
#29422=AXIS2_PLACEMENT_3D('',#127421,#33715,#33716);
#29423=AXIS2_PLACEMENT_3D('',#127427,#33720,#33721);
#29424=AXIS2_PLACEMENT_3D('',#127429,#33722,#33723);
#29425=AXIS2_PLACEMENT_3D('',#127431,#33724,#33725);
#29426=AXIS2_PLACEMENT_3D('',#127433,#33727,#33728);
#29427=AXIS2_PLACEMENT_3D('',#127439,#33732,#33733);
#29428=AXIS2_PLACEMENT_3D('',#127445,#33737,#33738);
#29429=AXIS2_PLACEMENT_3D('',#127448,#33741,#33742);
#29430=AXIS2_PLACEMENT_3D('',#127449,#33743,#33744);
#29431=AXIS2_PLACEMENT_3D('',#127450,#33745,#33746);
#29432=AXIS2_PLACEMENT_3D('',#127451,#33747,#33748);
#31762=DIRECTION('axis',(0.,0.,1.));
#31763=DIRECTION('refdir',(1.,0.,0.));
#32904=DIRECTION('center_axis',(-3.56963957938316E-5,-0.999999999362884,
0.));
#32905=DIRECTION('ref_axis',(0.,0.,-1.));
#32906=DIRECTION('center_axis',(0.,-1.,0.));
#32907=DIRECTION('ref_axis',(1.,0.,0.));
#32908=DIRECTION('center_axis',(-3.56963971012317E-5,-0.999999999362884,
0.));
#32909=DIRECTION('ref_axis',(0.,0.,-1.));
#32910=DIRECTION('',(-3.56963957938316E-5,-0.999999999362884,0.));
#32911=DIRECTION('center_axis',(-3.56963957938316E-5,-0.999999999362884,
0.));
#32912=DIRECTION('ref_axis',(0.,0.,-1.));
#32913=DIRECTION('center_axis',(3.56963957938316E-5,0.999999999362884,0.));
#32914=DIRECTION('ref_axis',(0.,0.,-1.));
#32915=DIRECTION('center_axis',(-3.56963957938316E-5,-0.999999999362884,
0.));
#32916=DIRECTION('ref_axis',(0.,0.,-1.));
#32917=DIRECTION('center_axis',(0.,-1.,0.));
#32918=DIRECTION('ref_axis',(1.,0.,0.));
#32919=DIRECTION('center_axis',(-3.56963971012317E-5,-0.999999999362884,
0.));
#32920=DIRECTION('ref_axis',(0.,0.,-1.));
#32921=DIRECTION('',(-3.56963957938316E-5,-0.999999999362884,0.));
#32922=DIRECTION('center_axis',(-3.56963957938316E-5,-0.999999999362884,
0.));
#32923=DIRECTION('ref_axis',(0.,0.,-1.));
#32924=DIRECTION('center_axis',(3.56963957938316E-5,0.999999999362884,0.));
#32925=DIRECTION('ref_axis',(0.,0.,-1.));
#32926=DIRECTION('center_axis',(0.,1.,0.));
#32927=DIRECTION('ref_axis',(-1.,0.,0.));
#32928=DIRECTION('',(0.,0.,1.));
#32929=DIRECTION('',(0.,0.,1.));
#32930=DIRECTION('',(-1.,0.,0.));
#32931=DIRECTION('',(0.,0.,1.));
#32932=DIRECTION('',(-1.,0.,0.));
#32933=DIRECTION('',(0.,0.,1.));
#32934=DIRECTION('center_axis',(-0.999999999362884,3.56963971012317E-5,
0.));
#32935=DIRECTION('ref_axis',(0.,0.,1.));
#32936=DIRECTION('',(0.,0.,1.));
#32937=DIRECTION('center_axis',(0.999999999362884,-3.56963971012317E-5,
0.));
#32938=DIRECTION('ref_axis',(0.,0.,1.));
#32939=DIRECTION('center_axis',(0.999999999362884,-3.56963971012835E-5,
0.));
#32940=DIRECTION('ref_axis',(0.,0.,1.));
#32941=DIRECTION('center_axis',(0.999999999362884,-3.56963971012317E-5,
0.));
#32942=DIRECTION('ref_axis',(0.,0.,1.));
#32943=DIRECTION('',(0.999999999362884,-3.56963971012835E-5,0.));
#32944=DIRECTION('center_axis',(-0.999999999362884,3.56963971012317E-5,
0.));
#32945=DIRECTION('ref_axis',(0.,0.,1.));
#32946=DIRECTION('',(-0.999999999362884,3.56963971012835E-5,0.));
#32947=DIRECTION('',(0.999999999362884,-3.56963971012835E-5,0.));
#32948=DIRECTION('center_axis',(-0.999999999362884,3.56963971012317E-5,
0.));
#32949=DIRECTION('ref_axis',(0.,0.,1.));
#32950=DIRECTION('center_axis',(-0.707132021900494,-0.707081539571582,0.));
#32951=DIRECTION('ref_axis',(0.707081539571582,-0.707132021900494,0.));
#32952=DIRECTION('',(-0.999999999362884,3.56963971012835E-5,0.));
#32953=DIRECTION('center_axis',(0.707081539571582,-0.707132021900494,0.));
#32954=DIRECTION('ref_axis',(-0.707132021900494,-0.707081539571582,0.));
#32955=DIRECTION('',(0.999999999362884,-3.56963971012835E-5,0.));
#32956=DIRECTION('',(-0.999999999362884,3.56963971012835E-5,0.));
#32957=DIRECTION('center_axis',(0.707081539571582,-0.707132021900494,0.));
#32958=DIRECTION('ref_axis',(-0.707132021900494,-0.707081539571582,0.));
#32959=DIRECTION('',(0.999999999362884,-3.56963971012835E-5,0.));
#32960=DIRECTION('center_axis',(-0.707106781186546,-0.707106781186549,0.));
#32961=DIRECTION('ref_axis',(0.707106781186549,-0.707106781186546,0.));
#32962=DIRECTION('',(-0.999999996715682,-1.14900183283708E-14,-8.104711771334E-5));
#32963=DIRECTION('',(0.999999996715682,1.14900183283708E-14,-8.104711771334E-5));
#32964=DIRECTION('center_axis',(-0.707106781186546,-0.707106781186549,0.));
#32965=DIRECTION('ref_axis',(0.707106781186549,-0.707106781186546,0.));
#32966=DIRECTION('',(-0.999999999639016,-4.22740799323897E-15,-2.68694483879996E-5));
#32967=DIRECTION('center_axis',(0.707106781186549,-0.707106781186546,0.));
#32968=DIRECTION('ref_axis',(-0.707106781186546,-0.707106781186549,0.));
#32969=DIRECTION('center_axis',(1.,0.,0.));
#32970=DIRECTION('ref_axis',(0.,-1.,0.));
#32971=DIRECTION('',(0.999999996701292,0.,-8.12244748976037E-5));
#32972=DIRECTION('',(-0.999999996701292,0.,-8.12244748976037E-5));
#32973=DIRECTION('center_axis',(1.,0.,0.));
#32974=DIRECTION('ref_axis',(0.,-1.,0.));
#32975=DIRECTION('',(0.999999999362884,-3.56963971012835E-5,0.));
#32976=DIRECTION('center_axis',(-1.,0.,0.));
#32977=DIRECTION('ref_axis',(0.,-1.,0.));
#32978=DIRECTION('center_axis',(-1.,0.,0.));
#32979=DIRECTION('ref_axis',(0.,-1.,0.));
#32980=DIRECTION('center_axis',(0.707106781186549,-0.707106781186546,0.));
#32981=DIRECTION('ref_axis',(-0.707106781186546,-0.707106781186549,0.));
#32982=DIRECTION('',(0.999999999639016,4.22740799323897E-15,-2.68694483879996E-5));
#32983=DIRECTION('center_axis',(-0.707106781186546,-0.707106781186549,0.));
#32984=DIRECTION('ref_axis',(0.707106781186549,-0.707106781186546,0.));
#32985=DIRECTION('center_axis',(0.707081539571582,-0.707132021900494,0.));
#32986=DIRECTION('ref_axis',(-0.707132021900494,-0.707081539571582,0.));
#32987=DIRECTION('',(0.999999999362884,-3.56963971012835E-5,0.));
#32988=DIRECTION('center_axis',(-0.707132021900494,-0.707081539571582,0.));
#32989=DIRECTION('ref_axis',(0.707081539571582,-0.707132021900494,0.));
#32990=DIRECTION('center_axis',(-0.999999999362884,3.56963971012317E-5,
0.));
#32991=DIRECTION('ref_axis',(0.,0.,1.));
#32992=DIRECTION('',(0.,0.,1.));
#32993=DIRECTION('center_axis',(0.999999999362884,-3.56963971012317E-5,
0.));
#32994=DIRECTION('ref_axis',(0.,0.,1.));
#32995=DIRECTION('center_axis',(0.999999999362884,-3.56963971012835E-5,
0.));
#32996=DIRECTION('ref_axis',(0.,0.,1.));
#32997=DIRECTION('center_axis',(0.999999999362884,-3.56963971012317E-5,
0.));
#32998=DIRECTION('ref_axis',(0.,0.,1.));
#32999=DIRECTION('',(0.999999999362884,-3.56963971012835E-5,0.));
#33000=DIRECTION('center_axis',(-0.999999999362884,3.56963971012317E-5,
0.));
#33001=DIRECTION('ref_axis',(0.,0.,1.));
#33002=DIRECTION('',(-0.999999999362884,3.56963971012835E-5,0.));
#33003=DIRECTION('',(0.999999999362884,-3.56963971012835E-5,0.));
#33004=DIRECTION('center_axis',(-0.999999999362884,3.56963971012317E-5,
0.));
#33005=DIRECTION('ref_axis',(0.,0.,1.));
#33006=DIRECTION('center_axis',(-0.707132021900494,-0.707081539571582,0.));
#33007=DIRECTION('ref_axis',(0.707081539571582,-0.707132021900494,0.));
#33008=DIRECTION('',(-0.999999999362884,3.56963971012835E-5,0.));
#33009=DIRECTION('center_axis',(0.707081539571582,-0.707132021900494,0.));
#33010=DIRECTION('ref_axis',(-0.707132021900494,-0.707081539571582,0.));
#33011=DIRECTION('',(0.999999999362884,-3.56963971012835E-5,0.));
#33012=DIRECTION('',(-0.999999999362884,3.56963971012835E-5,0.));
#33013=DIRECTION('center_axis',(0.707081539571582,-0.707132021900494,0.));
#33014=DIRECTION('ref_axis',(-0.707132021900494,-0.707081539571582,0.));
#33015=DIRECTION('',(0.999999999362884,-3.56963971012835E-5,0.));
#33016=DIRECTION('center_axis',(-0.707106781186546,-0.707106781186549,0.));
#33017=DIRECTION('ref_axis',(0.707106781186549,-0.707106781186546,0.));
#33018=DIRECTION('',(-0.999999996715682,-1.14900183283708E-14,-8.104711771334E-5));
#33019=DIRECTION('',(0.999999996715682,1.14900183283708E-14,-8.104711771334E-5));
#33020=DIRECTION('center_axis',(-0.707106781186546,-0.707106781186549,0.));
#33021=DIRECTION('ref_axis',(0.707106781186549,-0.707106781186546,0.));
#33022=DIRECTION('',(-0.999999999639016,-4.22740799323897E-15,-2.68694483879996E-5));
#33023=DIRECTION('center_axis',(0.707106781186549,-0.707106781186546,0.));
#33024=DIRECTION('ref_axis',(-0.707106781186546,-0.707106781186549,0.));
#33025=DIRECTION('center_axis',(1.,0.,0.));
#33026=DIRECTION('ref_axis',(0.,-1.,0.));
#33027=DIRECTION('',(0.999999996701292,0.,-8.12244748976037E-5));
#33028=DIRECTION('',(-0.999999996701292,0.,-8.12244748976037E-5));
#33029=DIRECTION('center_axis',(1.,0.,0.));
#33030=DIRECTION('ref_axis',(0.,-1.,0.));
#33031=DIRECTION('',(0.999999999362884,-3.56963971012835E-5,0.));
#33032=DIRECTION('center_axis',(-1.,0.,0.));
#33033=DIRECTION('ref_axis',(0.,-1.,0.));
#33034=DIRECTION('center_axis',(-1.,0.,0.));
#33035=DIRECTION('ref_axis',(0.,-1.,0.));
#33036=DIRECTION('center_axis',(0.707106781186549,-0.707106781186546,0.));
#33037=DIRECTION('ref_axis',(-0.707106781186546,-0.707106781186549,0.));
#33038=DIRECTION('',(0.999999999639016,4.22740799323897E-15,-2.68694483879996E-5));
#33039=DIRECTION('center_axis',(-0.707106781186546,-0.707106781186549,0.));
#33040=DIRECTION('ref_axis',(0.707106781186549,-0.707106781186546,0.));
#33041=DIRECTION('center_axis',(0.707081539571582,-0.707132021900494,0.));
#33042=DIRECTION('ref_axis',(-0.707132021900494,-0.707081539571582,0.));
#33043=DIRECTION('',(0.999999999362884,-3.56963971012835E-5,0.));
#33044=DIRECTION('center_axis',(-0.707132021900494,-0.707081539571582,0.));
#33045=DIRECTION('ref_axis',(0.707081539571582,-0.707132021900494,0.));
#33046=DIRECTION('center_axis',(-0.999999999362884,3.56963971012317E-5,
0.));
#33047=DIRECTION('ref_axis',(0.,0.,1.));
#33048=DIRECTION('',(0.,0.,1.));
#33049=DIRECTION('center_axis',(0.999999999362884,-3.56963971012317E-5,
0.));
#33050=DIRECTION('ref_axis',(0.,0.,1.));
#33051=DIRECTION('center_axis',(0.999999999362884,-3.56963971012835E-5,
0.));
#33052=DIRECTION('ref_axis',(0.,0.,1.));
#33053=DIRECTION('center_axis',(0.999999999362884,-3.56963971012317E-5,
0.));
#33054=DIRECTION('ref_axis',(0.,0.,1.));
#33055=DIRECTION('',(0.999999999362884,-3.56963971012835E-5,0.));
#33056=DIRECTION('center_axis',(-0.999999999362884,3.56963971012317E-5,
0.));
#33057=DIRECTION('ref_axis',(0.,0.,1.));
#33058=DIRECTION('',(-0.999999999362884,3.56963971012835E-5,0.));
#33059=DIRECTION('',(0.999999999362884,-3.56963971012835E-5,0.));
#33060=DIRECTION('center_axis',(-0.999999999362884,3.56963971012317E-5,
0.));
#33061=DIRECTION('ref_axis',(0.,0.,1.));
#33062=DIRECTION('center_axis',(-0.707132021900494,-0.707081539571582,0.));
#33063=DIRECTION('ref_axis',(0.707081539571582,-0.707132021900494,0.));
#33064=DIRECTION('',(-0.999999999362884,3.56963971012835E-5,0.));
#33065=DIRECTION('center_axis',(0.707081539571582,-0.707132021900494,0.));
#33066=DIRECTION('ref_axis',(-0.707132021900494,-0.707081539571582,0.));
#33067=DIRECTION('',(0.999999999362884,-3.56963971012835E-5,0.));
#33068=DIRECTION('',(-0.999999999362884,3.56963971012835E-5,0.));
#33069=DIRECTION('center_axis',(0.707081539571582,-0.707132021900494,0.));
#33070=DIRECTION('ref_axis',(-0.707132021900494,-0.707081539571582,0.));
#33071=DIRECTION('',(0.999999999362884,-3.56963971012835E-5,0.));
#33072=DIRECTION('center_axis',(-0.707106781186546,-0.707106781186549,0.));
#33073=DIRECTION('ref_axis',(0.707106781186549,-0.707106781186546,0.));
#33074=DIRECTION('',(-0.999999996715682,-1.14900183283708E-14,-8.10471177095101E-5));
#33075=DIRECTION('',(0.999999996715682,1.14900183283708E-14,-8.10471177095101E-5));
#33076=DIRECTION('center_axis',(-0.707106781186546,-0.707106781186549,0.));
#33077=DIRECTION('ref_axis',(0.707106781186549,-0.707106781186546,0.));
#33078=DIRECTION('',(-0.999999999639016,-4.22740799323898E-15,-2.6869448392227E-5));
#33079=DIRECTION('center_axis',(0.707106781186549,-0.707106781186546,0.));
#33080=DIRECTION('ref_axis',(-0.707106781186546,-0.707106781186549,0.));
#33081=DIRECTION('center_axis',(1.,0.,0.));
#33082=DIRECTION('ref_axis',(0.,-1.,0.));
#33083=DIRECTION('',(0.999999996701292,0.,-8.12244748976037E-5));
#33084=DIRECTION('',(-0.999999996701292,0.,-8.12244748976037E-5));
#33085=DIRECTION('center_axis',(1.,0.,0.));
#33086=DIRECTION('ref_axis',(0.,-1.,0.));
#33087=DIRECTION('',(0.999999999362884,-3.56963971012835E-5,0.));
#33088=DIRECTION('center_axis',(-1.,0.,0.));
#33089=DIRECTION('ref_axis',(0.,-1.,0.));
#33090=DIRECTION('center_axis',(-1.,0.,0.));
#33091=DIRECTION('ref_axis',(0.,-1.,0.));
#33092=DIRECTION('center_axis',(0.707106781186549,-0.707106781186546,0.));
#33093=DIRECTION('ref_axis',(-0.707106781186546,-0.707106781186549,0.));
#33094=DIRECTION('',(0.999999999639016,4.22740799323898E-15,-2.6869448392227E-5));
#33095=DIRECTION('center_axis',(-0.707106781186546,-0.707106781186549,0.));
#33096=DIRECTION('ref_axis',(0.707106781186549,-0.707106781186546,0.));
#33097=DIRECTION('center_axis',(0.707081539571582,-0.707132021900494,0.));
#33098=DIRECTION('ref_axis',(-0.707132021900494,-0.707081539571582,0.));
#33099=DIRECTION('',(0.999999999362884,-3.56963971012835E-5,0.));
#33100=DIRECTION('center_axis',(-0.707132021900494,-0.707081539571582,0.));
#33101=DIRECTION('ref_axis',(0.707081539571582,-0.707132021900494,0.));
#33102=DIRECTION('center_axis',(0.,0.,-1.));
#33103=DIRECTION('ref_axis',(0.999999999362884,-3.56963971012317E-5,0.));
#33104=DIRECTION('',(0.,0.,1.));
#33105=DIRECTION('center_axis',(0.,0.,-1.));
#33106=DIRECTION('ref_axis',(0.999999999362884,-3.56963971012317E-5,0.));
#33107=DIRECTION('',(0.,0.,1.));
#33108=DIRECTION('center_axis',(0.,0.,-1.));
#33109=DIRECTION('ref_axis',(0.999999999362884,-3.56963971012317E-5,0.));
#33110=DIRECTION('',(0.,0.,1.));
#33111=DIRECTION('',(0.,0.,1.));
#33112=DIRECTION('',(0.,0.,1.));
#33113=DIRECTION('center_axis',(3.56963971012317E-5,0.999999999362884,0.));
#33114=DIRECTION('ref_axis',(-0.999999999362884,3.56963971012317E-5,0.));
#33115=DIRECTION('',(0.,0.,1.));
#33116=DIRECTION('',(-0.999999999362884,3.56963971012317E-5,0.));
#33117=DIRECTION('center_axis',(3.56963971012317E-5,0.999999999362884,0.));
#33118=DIRECTION('ref_axis',(-0.999999999362884,3.56963971012317E-5,0.));
#33119=DIRECTION('',(-0.999999999362884,3.56963971012317E-5,0.));
#33120=DIRECTION('',(0.,0.,1.));
#33121=DIRECTION('center_axis',(3.56963971012317E-5,0.999999999362884,0.));
#33122=DIRECTION('ref_axis',(-0.999999999362884,3.56963971012317E-5,0.));
#33123=DIRECTION('',(0.,0.,1.));
#33124=DIRECTION('center_axis',(0.,0.,-1.));
#33125=DIRECTION('ref_axis',(-0.999999999362884,3.56963971012317E-5,0.));
#33126=DIRECTION('',(0.,0.,1.));
#33127=DIRECTION('center_axis',(0.,0.,-1.));
#33128=DIRECTION('ref_axis',(-0.999999999362884,3.56963971012317E-5,0.));
#33129=DIRECTION('center_axis',(0.,0.,-1.));
#33130=DIRECTION('ref_axis',(-0.999999999362884,3.56963971012317E-5,0.));
#33131=DIRECTION('center_axis',(0.,0.,1.));
#33132=DIRECTION('ref_axis',(-0.999999999362884,3.56963971012317E-5,0.));
#33133=DIRECTION('',(0.,0.,1.));
#33134=DIRECTION('center_axis',(0.,0.,-1.));
#33135=DIRECTION('ref_axis',(-0.999999999362884,3.56963971012317E-5,0.));
#33136=DIRECTION('',(0.,0.,1.));
#33137=DIRECTION('center_axis',(-0.999999999362884,3.56963971012317E-5,
0.));
#33138=DIRECTION('ref_axis',(-3.56963971012317E-5,-0.999999999362884,0.));
#33139=DIRECTION('',(0.,0.,1.));
#33140=DIRECTION('',(-3.56963971012317E-5,-0.999999999362884,0.));
#33141=DIRECTION('center_axis',(-0.999999999362884,3.56963971012317E-5,
0.));
#33142=DIRECTION('ref_axis',(-3.56963971012317E-5,-0.999999999362884,0.));
#33143=DIRECTION('',(-3.56963971012317E-5,-0.999999999362884,0.));
#33144=DIRECTION('',(0.,0.,1.));
#33145=DIRECTION('center_axis',(-0.999999999362884,3.56963971012317E-5,
0.));
#33146=DIRECTION('ref_axis',(-3.56963971012317E-5,-0.999999999362884,0.));
#33147=DIRECTION('',(0.,0.,1.));
#33148=DIRECTION('center_axis',(0.,0.,-1.));
#33149=DIRECTION('ref_axis',(-0.707132021900495,-0.707081539571582,0.));
#33150=DIRECTION('',(0.,0.,1.));
#33151=DIRECTION('center_axis',(0.,0.,-1.));
#33152=DIRECTION('ref_axis',(-0.707132021900495,-0.707081539571582,0.));
#33153=DIRECTION('center_axis',(0.,0.,-1.));
#33154=DIRECTION('ref_axis',(-0.707132021900495,-0.707081539571582,0.));
#33155=DIRECTION('center_axis',(0.,0.,1.));
#33156=DIRECTION('ref_axis',(-0.707132021900495,-0.707081539571582,0.));
#33157=DIRECTION('',(0.,0.,1.));
#33158=DIRECTION('center_axis',(0.,0.,-1.));
#33159=DIRECTION('ref_axis',(-0.707132021900495,-0.707081539571582,0.));
#33160=DIRECTION('',(0.,0.,1.));
#33161=DIRECTION('center_axis',(-0.707132021900494,-0.707081539571582,0.));
#33162=DIRECTION('ref_axis',(0.707081539571582,-0.707132021900494,0.));
#33163=DIRECTION('',(0.,0.,1.));
#33164=DIRECTION('',(0.707081539571582,-0.707132021900494,0.));
#33165=DIRECTION('center_axis',(-0.707132021900494,-0.707081539571582,0.));
#33166=DIRECTION('ref_axis',(0.707081539571582,-0.707132021900494,0.));
#33167=DIRECTION('',(0.707081539571582,-0.707132021900494,0.));
#33168=DIRECTION('',(0.,0.,1.));
#33169=DIRECTION('center_axis',(-0.707132021900494,-0.707081539571582,0.));
#33170=DIRECTION('ref_axis',(0.707081539571582,-0.707132021900494,0.));
#33171=DIRECTION('',(0.,0.,1.));
#33172=DIRECTION('center_axis',(0.,0.,-1.));
#33173=DIRECTION('ref_axis',(-3.56963971045624E-5,-0.999999999362884,0.));
#33174=DIRECTION('',(0.,0.,1.));
#33175=DIRECTION('center_axis',(0.,0.,-1.));
#33176=DIRECTION('ref_axis',(-3.56963971045624E-5,-0.999999999362884,0.));
#33177=DIRECTION('center_axis',(0.,0.,-1.));
#33178=DIRECTION('ref_axis',(-3.56963971045624E-5,-0.999999999362884,0.));
#33179=DIRECTION('center_axis',(0.,0.,1.));
#33180=DIRECTION('ref_axis',(-3.56963971045624E-5,-0.999999999362884,0.));
#33181=DIRECTION('',(0.,0.,1.));
#33182=DIRECTION('center_axis',(0.,0.,-1.));
#33183=DIRECTION('ref_axis',(-3.56963971045624E-5,-0.999999999362884,0.));
#33184=DIRECTION('',(0.,0.,1.));
#33185=DIRECTION('center_axis',(-3.56963971054591E-5,-0.999999999362884,
0.));
#33186=DIRECTION('ref_axis',(0.999999999362884,-3.56963971054591E-5,0.));
#33187=DIRECTION('',(0.,0.,1.));
#33188=DIRECTION('',(0.999999999362884,-3.56963971054591E-5,0.));
#33189=DIRECTION('center_axis',(-3.56963971054591E-5,-0.999999999362884,
0.));
#33190=DIRECTION('ref_axis',(0.999999999362884,-3.56963971054591E-5,0.));
#33191=DIRECTION('',(0.999999999362884,-3.56963971054591E-5,0.));
#33192=DIRECTION('',(0.,0.,1.));
#33193=DIRECTION('center_axis',(-3.56963971054591E-5,-0.999999999362884,
0.));
#33194=DIRECTION('ref_axis',(0.999999999362884,-3.56963971054591E-5,0.));
#33195=DIRECTION('',(0.,0.,1.));
#33196=DIRECTION('center_axis',(0.,0.,-1.));
#33197=DIRECTION('ref_axis',(0.707081539571582,-0.707132021900495,0.));
#33198=DIRECTION('',(0.,0.,1.));
#33199=DIRECTION('center_axis',(0.,0.,-1.));
#33200=DIRECTION('ref_axis',(0.707081539571582,-0.707132021900495,0.));
#33201=DIRECTION('center_axis',(0.,0.,-1.));
#33202=DIRECTION('ref_axis',(0.707081539571582,-0.707132021900495,0.));
#33203=DIRECTION('center_axis',(0.,0.,1.));
#33204=DIRECTION('ref_axis',(0.707081539571582,-0.707132021900495,0.));
#33205=DIRECTION('',(0.,0.,1.));
#33206=DIRECTION('center_axis',(0.,0.,-1.));
#33207=DIRECTION('ref_axis',(0.707081539571582,-0.707132021900495,0.));
#33208=DIRECTION('',(0.,0.,1.));
#33209=DIRECTION('center_axis',(0.707081539571582,-0.707132021900494,0.));
#33210=DIRECTION('ref_axis',(0.707132021900494,0.707081539571582,0.));
#33211=DIRECTION('',(0.,0.,1.));
#33212=DIRECTION('',(0.707132021900494,0.707081539571582,0.));
#33213=DIRECTION('center_axis',(0.707081539571582,-0.707132021900494,0.));
#33214=DIRECTION('ref_axis',(0.707132021900494,0.707081539571582,0.));
#33215=DIRECTION('',(0.707132021900494,0.707081539571582,0.));
#33216=DIRECTION('',(0.,0.,1.));
#33217=DIRECTION('center_axis',(0.707081539571582,-0.707132021900494,0.));
#33218=DIRECTION('ref_axis',(0.707132021900494,0.707081539571582,0.));
#33219=DIRECTION('',(0.,0.,1.));
#33220=DIRECTION('center_axis',(0.,0.,-1.));
#33221=DIRECTION('ref_axis',(3.56963971074767E-5,0.999999999362884,0.));
#33222=DIRECTION('',(0.,0.,1.));
#33223=DIRECTION('center_axis',(0.,0.,-1.));
#33224=DIRECTION('ref_axis',(3.56963971074767E-5,0.999999999362884,0.));
#33225=DIRECTION('center_axis',(0.,0.,-1.));
#33226=DIRECTION('ref_axis',(3.56963971074767E-5,0.999999999362884,0.));
#33227=DIRECTION('center_axis',(0.,0.,1.));
#33228=DIRECTION('ref_axis',(3.56963971074767E-5,0.999999999362884,0.));
#33229=DIRECTION('',(0.,0.,1.));
#33230=DIRECTION('center_axis',(0.,0.,-1.));
#33231=DIRECTION('ref_axis',(3.56963971074767E-5,0.999999999362884,0.));
#33232=DIRECTION('',(0.,0.,1.));
#33233=DIRECTION('center_axis',(3.56963971088917E-5,0.999999999362884,0.));
#33234=DIRECTION('ref_axis',(-0.999999999362884,3.56963971088917E-5,0.));
#33235=DIRECTION('',(0.,0.,1.));
#33236=DIRECTION('',(-0.999999999362884,3.56963971088917E-5,0.));
#33237=DIRECTION('center_axis',(3.56963971088917E-5,0.999999999362884,0.));
#33238=DIRECTION('ref_axis',(-0.999999999362884,3.56963971088917E-5,0.));
#33239=DIRECTION('',(-0.999999999362884,3.56963971088917E-5,0.));
#33240=DIRECTION('',(0.,0.,1.));
#33241=DIRECTION('center_axis',(3.56963971088917E-5,0.999999999362884,0.));
#33242=DIRECTION('ref_axis',(-0.999999999362884,3.56963971088917E-5,0.));
#33243=DIRECTION('',(0.,0.,1.));
#33244=DIRECTION('center_axis',(0.,0.,1.));
#33245=DIRECTION('ref_axis',(-1.,0.,0.));
#33246=DIRECTION('',(0.,0.,1.));
#33247=DIRECTION('',(0.,0.,1.));
#33248=DIRECTION('',(0.,0.,1.));
#33249=DIRECTION('center_axis',(0.,0.,1.));
#33250=DIRECTION('ref_axis',(-1.,0.,0.));
#33251=DIRECTION('',(0.,0.,1.));
#33252=DIRECTION('center_axis',(0.,0.,1.));
#33253=DIRECTION('ref_axis',(-1.,0.,0.));
#33254=DIRECTION('',(0.,0.,1.));
#33255=DIRECTION('center_axis',(0.,-1.,0.));
#33256=DIRECTION('ref_axis',(1.,0.,0.));
#33257=DIRECTION('',(0.,0.,1.));
#33258=DIRECTION('',(1.,0.,0.));
#33259=DIRECTION('center_axis',(0.,-1.,0.));
#33260=DIRECTION('ref_axis',(1.,0.,0.));
#33261=DIRECTION('',(0.,0.,1.));
#33262=DIRECTION('center_axis',(0.,-1.,0.));
#33263=DIRECTION('ref_axis',(1.,0.,0.));
#33264=DIRECTION('',(0.,0.,1.));
#33265=DIRECTION('center_axis',(0.,0.,1.));
#33266=DIRECTION('ref_axis',(1.,0.,0.));
#33267=DIRECTION('',(0.,0.,1.));
#33268=DIRECTION('center_axis',(0.,0.,-1.));
#33269=DIRECTION('ref_axis',(1.,0.,0.));
#33270=DIRECTION('center_axis',(0.,0.,1.));
#33271=DIRECTION('ref_axis',(1.,0.,0.));
#33272=DIRECTION('',(0.,0.,1.));
#33273=DIRECTION('center_axis',(0.,0.,1.));
#33274=DIRECTION('ref_axis',(1.,0.,0.));
#33275=DIRECTION('',(0.,0.,1.));
#33276=DIRECTION('center_axis',(-1.,0.,0.));
#33277=DIRECTION('ref_axis',(0.,-1.,0.));
#33278=DIRECTION('',(0.,0.,1.));
#33279=DIRECTION('',(0.,-1.,0.));
#33280=DIRECTION('center_axis',(-1.,0.,0.));
#33281=DIRECTION('ref_axis',(0.,-1.,0.));
#33282=DIRECTION('',(0.,0.,1.));
#33283=DIRECTION('center_axis',(-1.,0.,0.));
#33284=DIRECTION('ref_axis',(0.,-1.,0.));
#33285=DIRECTION('',(0.,0.,1.));
#33286=DIRECTION('center_axis',(0.,0.,1.));
#33287=DIRECTION('ref_axis',(0.70710678118655,-0.707106781186545,0.));
#33288=DIRECTION('',(0.,0.,1.));
#33289=DIRECTION('center_axis',(0.,0.,-1.));
#33290=DIRECTION('ref_axis',(0.70710678118655,-0.707106781186545,0.));
#33291=DIRECTION('center_axis',(0.,0.,1.));
#33292=DIRECTION('ref_axis',(0.70710678118655,-0.707106781186545,0.));
#33293=DIRECTION('',(0.,0.,1.));
#33294=DIRECTION('center_axis',(0.,0.,1.));
#33295=DIRECTION('ref_axis',(0.70710678118655,-0.707106781186545,0.));
#33296=DIRECTION('',(0.,0.,1.));
#33297=DIRECTION('center_axis',(-0.707106781186549,0.707106781186546,0.));
#33298=DIRECTION('ref_axis',(-0.707106781186546,-0.707106781186549,0.));
#33299=DIRECTION('',(0.,0.,1.));
#33300=DIRECTION('',(-0.707106781186546,-0.707106781186549,0.));
#33301=DIRECTION('center_axis',(-0.707106781186549,0.707106781186546,0.));
#33302=DIRECTION('ref_axis',(-0.707106781186546,-0.707106781186549,0.));
#33303=DIRECTION('',(0.,0.,1.));
#33304=DIRECTION('center_axis',(-0.707106781186549,0.707106781186546,0.));
#33305=DIRECTION('ref_axis',(-0.707106781186546,-0.707106781186549,0.));
#33306=DIRECTION('',(0.,0.,1.));
#33307=DIRECTION('center_axis',(0.,0.,1.));
#33308=DIRECTION('ref_axis',(3.33066907387547E-15,-1.,0.));
#33309=DIRECTION('',(0.,0.,1.));
#33310=DIRECTION('center_axis',(0.,0.,-1.));
#33311=DIRECTION('ref_axis',(3.33066907387547E-15,-1.,0.));
#33312=DIRECTION('center_axis',(0.,0.,1.));
#33313=DIRECTION('ref_axis',(3.33066907387547E-15,-1.,0.));
#33314=DIRECTION('',(0.,0.,1.));
#33315=DIRECTION('center_axis',(0.,0.,1.));
#33316=DIRECTION('ref_axis',(3.33066907387547E-15,-1.,0.));
#33317=DIRECTION('',(0.,0.,1.));
#33318=DIRECTION('center_axis',(-4.22740799476499E-15,1.,0.));
#33319=DIRECTION('ref_axis',(-1.,-4.22740799476499E-15,0.));
#33320=DIRECTION('',(0.,0.,1.));
#33321=DIRECTION('',(-1.,-4.22740799476499E-15,0.));
#33322=DIRECTION('center_axis',(-4.22740799476499E-15,1.,0.));
#33323=DIRECTION('ref_axis',(-1.,-4.22740799476499E-15,0.));
#33324=DIRECTION('',(0.,0.,1.));
#33325=DIRECTION('center_axis',(-4.22740799476499E-15,1.,0.));
#33326=DIRECTION('ref_axis',(-1.,-4.22740799476499E-15,0.));
#33327=DIRECTION('',(0.,0.,1.));
#33328=DIRECTION('center_axis',(0.,0.,1.));
#33329=DIRECTION('ref_axis',(-0.707106781186545,-0.70710678118655,0.));
#33330=DIRECTION('',(0.,0.,1.));
#33331=DIRECTION('center_axis',(0.,0.,-1.));
#33332=DIRECTION('ref_axis',(-0.707106781186545,-0.70710678118655,0.));
#33333=DIRECTION('center_axis',(0.,0.,1.));
#33334=DIRECTION('ref_axis',(-0.707106781186545,-0.70710678118655,0.));
#33335=DIRECTION('',(0.,0.,1.));
#33336=DIRECTION('center_axis',(0.,0.,1.));
#33337=DIRECTION('ref_axis',(-0.707106781186545,-0.70710678118655,0.));
#33338=DIRECTION('',(0.,0.,1.));
#33339=DIRECTION('center_axis',(0.707106781186546,0.707106781186549,0.));
#33340=DIRECTION('ref_axis',(-0.707106781186549,0.707106781186546,0.));
#33341=DIRECTION('',(0.,0.,1.));
#33342=DIRECTION('',(-0.707106781186549,0.707106781186546,0.));
#33343=DIRECTION('center_axis',(0.707106781186546,0.707106781186549,0.));
#33344=DIRECTION('ref_axis',(-0.707106781186549,0.707106781186546,0.));
#33345=DIRECTION('',(0.,0.,1.));
#33346=DIRECTION('center_axis',(0.707106781186546,0.707106781186549,0.));
#33347=DIRECTION('ref_axis',(-0.707106781186549,0.707106781186546,0.));
#33348=DIRECTION('',(0.,0.,1.));
#33349=DIRECTION('center_axis',(0.,0.,1.));
#33350=DIRECTION('ref_axis',(-6.2450045135165E-15,1.,0.));
#33351=DIRECTION('',(0.,0.,1.));
#33352=DIRECTION('center_axis',(0.,0.,-1.));
#33353=DIRECTION('ref_axis',(-6.2450045135165E-15,1.,0.));
#33354=DIRECTION('center_axis',(0.,0.,1.));
#33355=DIRECTION('ref_axis',(-6.2450045135165E-15,1.,0.));
#33356=DIRECTION('',(0.,0.,1.));
#33357=DIRECTION('center_axis',(0.,0.,1.));
#33358=DIRECTION('ref_axis',(-6.2450045135165E-15,1.,0.));
#33359=DIRECTION('',(0.,0.,1.));
#33360=DIRECTION('center_axis',(7.6600122440718E-15,-1.,0.));
#33361=DIRECTION('ref_axis',(1.,7.6600122440718E-15,0.));
#33362=DIRECTION('',(0.,0.,1.));
#33363=DIRECTION('',(1.,7.6600122440718E-15,0.));
#33364=DIRECTION('center_axis',(7.6600122440718E-15,-1.,0.));
#33365=DIRECTION('ref_axis',(1.,7.6600122440718E-15,0.));
#33366=DIRECTION('',(0.,0.,1.));
#33367=DIRECTION('center_axis',(7.6600122440718E-15,-1.,0.));
#33368=DIRECTION('ref_axis',(1.,7.6600122440718E-15,0.));
#33369=DIRECTION('',(0.,0.,1.));
#33370=DIRECTION('center_axis',(0.999999999362884,-3.56963971013892E-5,
0.));
#33371=DIRECTION('ref_axis',(0.,0.,1.));
#33372=DIRECTION('center_axis',(0.999999999362884,-3.56963971012317E-5,
0.));
#33373=DIRECTION('ref_axis',(0.,0.,1.));
#33374=DIRECTION('',(0.999999999362884,-3.56963971013892E-5,0.));
#33375=DIRECTION('center_axis',(-0.999999999362884,3.56963971012317E-5,
0.));
#33376=DIRECTION('ref_axis',(0.,0.,1.));
#33377=DIRECTION('center_axis',(0.999999999362884,-3.56963971013892E-5,
0.));
#33378=DIRECTION('ref_axis',(0.,0.,1.));
#33379=DIRECTION('center_axis',(0.999999999362884,-3.56963971012317E-5,
0.));
#33380=DIRECTION('ref_axis',(0.,0.,1.));
#33381=DIRECTION('',(0.999999999362884,-3.56963971013892E-5,0.));
#33382=DIRECTION('center_axis',(-0.999999999362884,3.56963971012317E-5,
0.));
#33383=DIRECTION('ref_axis',(0.,0.,1.));
#33384=DIRECTION('center_axis',(0.999999999362884,-3.56963971013892E-5,
0.));
#33385=DIRECTION('ref_axis',(0.,0.,1.));
#33386=DIRECTION('center_axis',(0.999999999362884,-3.56963971012317E-5,
0.));
#33387=DIRECTION('ref_axis',(0.,0.,1.));
#33388=DIRECTION('',(0.999999999362884,-3.56963971013892E-5,0.));
#33389=DIRECTION('center_axis',(-0.999999999362884,3.56963971012317E-5,
0.));
#33390=DIRECTION('ref_axis',(0.,0.,1.));
#33391=DIRECTION('center_axis',(3.56963971012317E-5,0.999999999362884,0.));
#33392=DIRECTION('ref_axis',(-0.999999999362884,3.56963971012317E-5,0.));
#33393=DIRECTION('',(0.999999999362884,-3.56963971012317E-5,0.));
#33394=DIRECTION('',(0.,0.,1.));
#33395=DIRECTION('',(-0.999999999362884,3.56963971012317E-5,0.));
#33396=DIRECTION('',(0.,0.,1.));
#33397=DIRECTION('center_axis',(-3.56963971012317E-5,-0.999999999362884,
0.));
#33398=DIRECTION('ref_axis',(0.999999999362884,-3.56963971012317E-5,0.));
#33399=DIRECTION('',(0.999999999362884,-3.56963971012317E-5,0.));
#33400=DIRECTION('',(0.,0.,1.));
#33401=DIRECTION('',(0.999999999362884,-3.56963971012317E-5,0.));
#33402=DIRECTION('center_axis',(0.,0.,-1.));
#33403=DIRECTION('ref_axis',(-0.999999999362884,3.56963971012317E-5,0.));
#33404=DIRECTION('center_axis',(0.,0.,-1.));
#33405=DIRECTION('ref_axis',(-0.999999999362884,3.56963971012317E-5,0.));
#33406=DIRECTION('',(0.,0.,1.));
#33407=DIRECTION('center_axis',(0.,0.,-1.));
#33408=DIRECTION('ref_axis',(-0.999999999362884,3.56963971012317E-5,0.));
#33409=DIRECTION('center_axis',(0.999999999362884,-3.56963971012317E-5,
0.));
#33410=DIRECTION('ref_axis',(3.56963971012317E-5,0.999999999362884,0.));
#33411=DIRECTION('',(3.56963971012317E-5,0.999999999362884,0.));
#33412=DIRECTION('',(0.,0.,1.));
#33413=DIRECTION('',(3.56963971012317E-5,0.999999999362884,0.));
#33414=DIRECTION('center_axis',(0.,0.,-1.));
#33415=DIRECTION('ref_axis',(-3.56963971086332E-5,-0.999999999362884,0.));
#33416=DIRECTION('',(0.,0.,1.));
#33417=DIRECTION('center_axis',(0.,0.,-1.));
#33418=DIRECTION('ref_axis',(-3.56963971086332E-5,-0.999999999362884,0.));
#33419=DIRECTION('center_axis',(0.,0.,-1.));
#33420=DIRECTION('ref_axis',(-3.56963971086332E-5,-0.999999999362884,0.));
#33421=DIRECTION('center_axis',(3.56963971088917E-5,0.999999999362884,0.));
#33422=DIRECTION('ref_axis',(-0.999999999362884,3.56963971088917E-5,0.));
#33423=DIRECTION('',(0.,0.,1.));
#33424=DIRECTION('center_axis',(0.,0.,-1.));
#33425=DIRECTION('ref_axis',(3.56963971074767E-5,0.999999999362884,0.));
#33426=DIRECTION('',(0.,0.,1.));
#33427=DIRECTION('center_axis',(0.707081539571582,-0.707132021900494,0.));
#33428=DIRECTION('ref_axis',(0.707132021900494,0.707081539571582,0.));
#33429=DIRECTION('',(0.,0.,1.));
#33430=DIRECTION('center_axis',(0.,0.,-1.));
#33431=DIRECTION('ref_axis',(0.707081539571582,-0.707132021900495,0.));
#33432=DIRECTION('',(0.,0.,1.));
#33433=DIRECTION('center_axis',(-3.56963971054591E-5,-0.999999999362884,
0.));
#33434=DIRECTION('ref_axis',(0.999999999362884,-3.56963971054591E-5,0.));
#33435=DIRECTION('',(0.,0.,1.));
#33436=DIRECTION('center_axis',(0.,0.,-1.));
#33437=DIRECTION('ref_axis',(-3.56963971045624E-5,-0.999999999362884,0.));
#33438=DIRECTION('',(0.,0.,1.));
#33439=DIRECTION('center_axis',(-0.707132021900494,-0.707081539571582,0.));
#33440=DIRECTION('ref_axis',(0.707081539571582,-0.707132021900494,0.));
#33441=DIRECTION('',(0.,0.,1.));
#33442=DIRECTION('center_axis',(0.,0.,-1.));
#33443=DIRECTION('ref_axis',(-0.707132021900495,-0.707081539571582,0.));
#33444=DIRECTION('',(0.,0.,1.));
#33445=DIRECTION('center_axis',(-0.999999999362884,3.56963971012317E-5,
0.));
#33446=DIRECTION('ref_axis',(-3.56963971012317E-5,-0.999999999362884,0.));
#33447=DIRECTION('',(0.,0.,1.));
#33448=DIRECTION('center_axis',(0.,0.,-1.));
#33449=DIRECTION('ref_axis',(-0.999999999362884,3.56963971012317E-5,0.));
#33450=DIRECTION('',(0.,0.,1.));
#33451=DIRECTION('center_axis',(3.56963971012317E-5,0.999999999362884,0.));
#33452=DIRECTION('ref_axis',(-0.999999999362884,3.56963971012317E-5,0.));
#33453=DIRECTION('center_axis',(-0.999999999362884,3.56963971012317E-5,
0.));
#33454=DIRECTION('ref_axis',(-3.56963971012317E-5,-0.999999999362884,0.));
#33455=DIRECTION('',(-3.56963971012317E-5,-0.999999999362884,0.));
#33456=DIRECTION('',(0.,0.,1.));
#33457=DIRECTION('',(-3.56963971012317E-5,-0.999999999362884,0.));
#33458=DIRECTION('center_axis',(0.,0.,-1.));
#33459=DIRECTION('ref_axis',(3.56963971012317E-5,0.999999999362884,0.));
#33460=DIRECTION('center_axis',(0.,0.,-1.));
#33461=DIRECTION('ref_axis',(3.56963971012317E-5,0.999999999362884,0.));
#33462=DIRECTION('',(0.,0.,1.));
#33463=DIRECTION('center_axis',(0.,0.,-1.));
#33464=DIRECTION('ref_axis',(3.56963971012317E-5,0.999999999362884,0.));
#33465=DIRECTION('center_axis',(-3.56963971012317E-5,-0.999999999362884,
0.));
#33466=DIRECTION('ref_axis',(0.999999999362884,-3.56963971012317E-5,0.));
#33467=DIRECTION('',(0.999999999362884,-3.56963971012317E-5,0.));
#33468=DIRECTION('',(0.,0.,1.));
#33469=DIRECTION('',(0.999999999362884,-3.56963971012317E-5,0.));
#33470=DIRECTION('center_axis',(0.,0.,-1.));
#33471=DIRECTION('ref_axis',(-0.999999999362884,3.56963971012317E-5,0.));
#33472=DIRECTION('center_axis',(0.,0.,-1.));
#33473=DIRECTION('ref_axis',(-0.999999999362884,3.56963971012317E-5,0.));
#33474=DIRECTION('',(0.,0.,1.));
#33475=DIRECTION('center_axis',(0.,0.,-1.));
#33476=DIRECTION('ref_axis',(-0.999999999362884,3.56963971012317E-5,0.));
#33477=DIRECTION('center_axis',(0.999999999362884,-3.56963971012317E-5,
0.));
#33478=DIRECTION('ref_axis',(3.56963971012317E-5,0.999999999362884,0.));
#33479=DIRECTION('',(3.56963971012317E-5,0.999999999362884,0.));
#33480=DIRECTION('',(0.,0.,1.));
#33481=DIRECTION('',(3.56963971012317E-5,0.999999999362884,0.));
#33482=DIRECTION('center_axis',(0.,0.,-1.));
#33483=DIRECTION('ref_axis',(0.999999999362884,-3.56963971012317E-5,0.));
#33484=DIRECTION('center_axis',(0.,0.,-1.));
#33485=DIRECTION('ref_axis',(0.999999999362884,-3.56963971012317E-5,0.));
#33486=DIRECTION('',(0.,0.,1.));
#33487=DIRECTION('center_axis',(0.,0.,1.));
#33488=DIRECTION('ref_axis',(0.999999999362884,-3.56963971012317E-5,0.));
#33489=DIRECTION('center_axis',(-3.56963971012317E-5,-0.999999999362884,
0.));
#33490=DIRECTION('ref_axis',(0.999999999362884,-3.56963971012317E-5,0.));
#33491=DIRECTION('',(0.999999999362884,-3.56963971012317E-5,0.));
#33492=DIRECTION('',(0.,0.,1.));
#33493=DIRECTION('',(0.999999999362884,-3.56963971012317E-5,0.));
#33494=DIRECTION('center_axis',(0.,0.,-1.));
#33495=DIRECTION('ref_axis',(-0.707081539571584,0.707132021900492,0.));
#33496=DIRECTION('center_axis',(0.,0.,-1.));
#33497=DIRECTION('ref_axis',(-0.707081539571584,0.707132021900492,0.));
#33498=DIRECTION('',(0.,0.,1.));
#33499=DIRECTION('center_axis',(0.,0.,-1.));
#33500=DIRECTION('ref_axis',(-0.707081539571584,0.707132021900492,0.));
#33501=DIRECTION('center_axis',(0.707081539571584,-0.707132021900493,0.));
#33502=DIRECTION('ref_axis',(0.707132021900493,0.707081539571584,0.));
#33503=DIRECTION('',(0.707132021900493,0.707081539571584,0.));
#33504=DIRECTION('',(0.,0.,1.));
#33505=DIRECTION('',(0.707132021900493,0.707081539571584,0.));
#33506=DIRECTION('center_axis',(0.,0.,-1.));
#33507=DIRECTION('ref_axis',(-0.999999999362884,3.56963971012317E-5,0.));
#33508=DIRECTION('center_axis',(0.,0.,-1.));
#33509=DIRECTION('ref_axis',(-0.999999999362884,3.56963971012317E-5,0.));
#33510=DIRECTION('',(0.,0.,1.));
#33511=DIRECTION('center_axis',(0.,0.,-1.));
#33512=DIRECTION('ref_axis',(-0.999999999362884,3.56963971012317E-5,0.));
#33513=DIRECTION('center_axis',(0.999999999362884,-3.56963971012317E-5,
0.));
#33514=DIRECTION('ref_axis',(3.56963971012317E-5,0.999999999362884,0.));
#33515=DIRECTION('',(3.56963971012317E-5,0.999999999362884,0.));
#33516=DIRECTION('',(0.,0.,1.));
#33517=DIRECTION('',(3.56963971012317E-5,0.999999999362884,0.));
#33518=DIRECTION('center_axis',(0.,0.,-1.));
#33519=DIRECTION('ref_axis',(-3.56963971012317E-5,-0.999999999362884,0.));
#33520=DIRECTION('center_axis',(0.,0.,-1.));
#33521=DIRECTION('ref_axis',(-3.56963971012317E-5,-0.999999999362884,0.));
#33522=DIRECTION('',(0.,0.,1.));
#33523=DIRECTION('center_axis',(0.,0.,-1.));
#33524=DIRECTION('ref_axis',(-3.56963971012317E-5,-0.999999999362884,0.));
#33525=DIRECTION('center_axis',(3.56963971012317E-5,0.999999999362884,0.));
#33526=DIRECTION('ref_axis',(-0.999999999362884,3.56963971012317E-5,0.));
#33527=DIRECTION('',(-0.999999999362884,3.56963971012317E-5,0.));
#33528=DIRECTION('',(0.,0.,1.));
#33529=DIRECTION('',(-0.999999999362884,3.56963971012317E-5,0.));
#33530=DIRECTION('center_axis',(-0.707081539571583,0.707132021900493,0.));
#33531=DIRECTION('ref_axis',(-0.707132021900493,-0.707081539571583,0.));
#33532=DIRECTION('',(-0.707132021900493,-0.707081539571583,0.));
#33533=DIRECTION('',(0.,0.,1.));
#33534=DIRECTION('',(-0.707132021900493,-0.707081539571583,0.));
#33535=DIRECTION('center_axis',(-0.999999999362884,3.56963971012317E-5,
0.));
#33536=DIRECTION('ref_axis',(-3.56963971012317E-5,-0.999999999362884,0.));
#33537=DIRECTION('',(-3.56963971012317E-5,-0.999999999362884,0.));
#33538=DIRECTION('',(0.,0.,1.));
#33539=DIRECTION('',(-3.56963971012317E-5,-0.999999999362884,0.));
#33540=DIRECTION('center_axis',(0.,0.,-1.));
#33541=DIRECTION('ref_axis',(-0.999999999362884,3.56963971012317E-5,0.));
#33542=DIRECTION('center_axis',(0.,0.,-1.));
#33543=DIRECTION('ref_axis',(-0.999999999362884,3.56963971012317E-5,0.));
#33544=DIRECTION('',(0.,0.,1.));
#33545=DIRECTION('center_axis',(0.,0.,1.));
#33546=DIRECTION('ref_axis',(-0.999999999362884,3.56963971012317E-5,0.));
#33547=DIRECTION('center_axis',(-0.469440044438888,0.88296435073972,0.));
#33548=DIRECTION('ref_axis',(-0.88296435073972,-0.469440044438888,0.));
#33549=DIRECTION('',(-0.88296435073972,-0.469440044438887,0.));
#33550=DIRECTION('',(0.,0.,1.));
#33551=DIRECTION('',(-0.88296435073972,-0.469440044438887,0.));
#33552=DIRECTION('center_axis',(3.56963971012317E-5,0.999999999362884,0.));
#33553=DIRECTION('ref_axis',(-0.999999999362884,3.56963971012317E-5,0.));
#33554=DIRECTION('',(-0.999999999362884,3.56963971012317E-5,0.));
#33555=DIRECTION('',(0.,0.,1.));
#33556=DIRECTION('',(-0.999999999362884,3.56963971012317E-5,0.));
#33557=DIRECTION('center_axis',(-0.999999999362884,3.56963971012317E-5,
0.));
#33558=DIRECTION('ref_axis',(-3.56963971012317E-5,-0.999999999362884,0.));
#33559=DIRECTION('',(-3.56963971012317E-5,-0.999999999362884,0.));
#33560=DIRECTION('',(-3.56963971012317E-5,-0.999999999362884,0.));
#33561=DIRECTION('center_axis',(0.,-1.,0.));
#33562=DIRECTION('ref_axis',(1.,0.,0.));
#33563=DIRECTION('',(-1.,0.,0.));
#33564=DIRECTION('',(0.,0.,1.));
#33565=DIRECTION('',(1.,0.,0.));
#33566=DIRECTION('center_axis',(0.,0.,1.));
#33567=DIRECTION('ref_axis',(1.,0.,0.));
#33568=DIRECTION('center_axis',(0.,0.,1.));
#33569=DIRECTION('ref_axis',(1.,0.,0.));
#33570=DIRECTION('center_axis',(0.,0.,1.));
#33571=DIRECTION('ref_axis',(1.,0.,0.));
#33572=DIRECTION('',(0.,0.,1.));
#33573=DIRECTION('center_axis',(1.,0.,0.));
#33574=DIRECTION('ref_axis',(0.,1.,0.));
#33575=DIRECTION('',(0.,1.,0.));
#33576=DIRECTION('',(0.,1.,0.));
#33577=DIRECTION('',(0.,0.,1.));
#33578=DIRECTION('center_axis',(0.,0.,1.));
#33579=DIRECTION('ref_axis',(7.40148683083432E-15,-1.,0.));
#33580=DIRECTION('',(0.,0.,1.));
#33581=DIRECTION('center_axis',(0.,0.,1.));
#33582=DIRECTION('ref_axis',(7.40148683083432E-15,-1.,0.));
#33583=DIRECTION('center_axis',(0.,0.,1.));
#33584=DIRECTION('ref_axis',(7.40148683083432E-15,-1.,0.));
#33585=DIRECTION('center_axis',(7.6600122440718E-15,-1.,0.));
#33586=DIRECTION('ref_axis',(1.,7.6600122440718E-15,0.));
#33587=DIRECTION('',(0.,0.,1.));
#33588=DIRECTION('',(1.,7.6600122440718E-15,0.));
#33589=DIRECTION('center_axis',(0.,0.,1.));
#33590=DIRECTION('ref_axis',(-6.2450045135165E-15,1.,0.));
#33591=DIRECTION('',(0.,0.,1.));
#33592=DIRECTION('center_axis',(0.,0.,1.));
#33593=DIRECTION('ref_axis',(-6.2450045135165E-15,1.,0.));
#33594=DIRECTION('center_axis',(0.707106781186546,0.707106781186549,0.));
#33595=DIRECTION('ref_axis',(-0.707106781186549,0.707106781186546,0.));
#33596=DIRECTION('',(0.,0.,1.));
#33597=DIRECTION('',(-0.707106781186549,0.707106781186546,0.));
#33598=DIRECTION('center_axis',(0.,0.,1.));
#33599=DIRECTION('ref_axis',(-0.707106781186545,-0.70710678118655,0.));
#33600=DIRECTION('',(0.,0.,1.));
#33601=DIRECTION('center_axis',(0.,0.,1.));
#33602=DIRECTION('ref_axis',(-0.707106781186545,-0.70710678118655,0.));
#33603=DIRECTION('center_axis',(-4.22740799476499E-15,1.,0.));
#33604=DIRECTION('ref_axis',(-1.,-4.22740799476499E-15,0.));
#33605=DIRECTION('',(0.,0.,1.));
#33606=DIRECTION('',(-1.,-4.22740799476499E-15,0.));
#33607=DIRECTION('center_axis',(0.,0.,1.));
#33608=DIRECTION('ref_axis',(3.33066907387547E-15,-1.,0.));
#33609=DIRECTION('',(0.,0.,1.));
#33610=DIRECTION('center_axis',(0.,0.,1.));
#33611=DIRECTION('ref_axis',(3.33066907387547E-15,-1.,0.));
#33612=DIRECTION('center_axis',(-0.707106781186549,0.707106781186546,0.));
#33613=DIRECTION('ref_axis',(-0.707106781186546,-0.707106781186549,0.));
#33614=DIRECTION('',(0.,0.,1.));
#33615=DIRECTION('',(-0.707106781186546,-0.707106781186549,0.));
#33616=DIRECTION('center_axis',(0.,0.,1.));
#33617=DIRECTION('ref_axis',(0.70710678118655,-0.707106781186545,0.));
#33618=DIRECTION('',(0.,0.,1.));
#33619=DIRECTION('center_axis',(0.,0.,1.));
#33620=DIRECTION('ref_axis',(0.70710678118655,-0.707106781186545,0.));
#33621=DIRECTION('center_axis',(-1.,0.,0.));
#33622=DIRECTION('ref_axis',(0.,-1.,0.));
#33623=DIRECTION('',(0.,0.,1.));
#33624=DIRECTION('',(0.,-1.,0.));
#33625=DIRECTION('center_axis',(0.,0.,1.));
#33626=DIRECTION('ref_axis',(1.,0.,0.));
#33627=DIRECTION('',(0.,0.,1.));
#33628=DIRECTION('center_axis',(0.,0.,1.));
#33629=DIRECTION('ref_axis',(1.,0.,0.));
#33630=DIRECTION('center_axis',(0.,-1.,0.));
#33631=DIRECTION('ref_axis',(1.,0.,0.));
#33632=DIRECTION('',(1.,0.,0.));
#33633=DIRECTION('center_axis',(-1.,0.,0.));
#33634=DIRECTION('ref_axis',(0.,-1.,0.));
#33635=DIRECTION('',(0.,-1.,0.));
#33636=DIRECTION('',(0.,-1.,0.));
#33637=DIRECTION('',(0.,0.,1.));
#33638=DIRECTION('center_axis',(0.,0.,1.));
#33639=DIRECTION('ref_axis',(0.,1.,0.));
#33640=DIRECTION('center_axis',(0.,0.,1.));
#33641=DIRECTION('ref_axis',(0.,1.,0.));
#33642=DIRECTION('center_axis',(0.,0.,1.));
#33643=DIRECTION('ref_axis',(0.,1.,0.));
#33644=DIRECTION('',(0.,0.,1.));
#33645=DIRECTION('center_axis',(0.,1.,0.));
#33646=DIRECTION('ref_axis',(-1.,0.,0.));
#33647=DIRECTION('',(-1.,0.,0.));
#33648=DIRECTION('',(-1.,0.,0.));
#33649=DIRECTION('',(0.,0.,1.));
#33650=DIRECTION('center_axis',(0.,0.,1.));
#33651=DIRECTION('ref_axis',(1.,0.,0.));
#33652=DIRECTION('center_axis',(0.,0.,1.));
#33653=DIRECTION('ref_axis',(1.,0.,0.));
#33654=DIRECTION('center_axis',(0.,0.,1.));
#33655=DIRECTION('ref_axis',(1.,0.,0.));
#33656=DIRECTION('',(0.,0.,1.));
#33657=DIRECTION('center_axis',(1.,0.,0.));
#33658=DIRECTION('ref_axis',(0.,1.,0.));
#33659=DIRECTION('',(0.,1.,0.));
#33660=DIRECTION('',(0.,1.,0.));
#33661=DIRECTION('',(0.,0.,1.));
#33662=DIRECTION('center_axis',(0.,0.,1.));
#33663=DIRECTION('ref_axis',(-1.,0.,0.));
#33664=DIRECTION('center_axis',(0.,0.,1.));
#33665=DIRECTION('ref_axis',(-1.,0.,0.));
#33666=DIRECTION('center_axis',(0.,0.,-1.));
#33667=DIRECTION('ref_axis',(-1.,0.,0.));
#33668=DIRECTION('',(0.,0.,1.));
#33669=DIRECTION('center_axis',(0.,1.,0.));
#33670=DIRECTION('ref_axis',(-1.,0.,0.));
#33671=DIRECTION('',(-1.,0.,0.));
#33672=DIRECTION('',(-1.,0.,0.));
#33673=DIRECTION('',(0.,0.,1.));
#33674=DIRECTION('center_axis',(0.,0.,1.));
#33675=DIRECTION('ref_axis',(0.707106781186548,0.707106781186547,0.));
#33676=DIRECTION('center_axis',(0.,0.,1.));
#33677=DIRECTION('ref_axis',(0.707106781186548,0.707106781186547,0.));
#33678=DIRECTION('center_axis',(0.,0.,1.));
#33679=DIRECTION('ref_axis',(0.707106781186548,0.707106781186547,0.));
#33680=DIRECTION('',(0.,0.,1.));
#33681=DIRECTION('center_axis',(0.707106781186547,0.707106781186548,0.));
#33682=DIRECTION('ref_axis',(-0.707106781186548,0.707106781186547,0.));
#33683=DIRECTION('',(-0.707106781186548,0.707106781186547,0.));
#33684=DIRECTION('',(-0.707106781186548,0.707106781186547,0.));
#33685=DIRECTION('',(0.,0.,1.));
#33686=DIRECTION('center_axis',(0.,0.,1.));
#33687=DIRECTION('ref_axis',(1.,0.,0.));
#33688=DIRECTION('center_axis',(0.,0.,1.));
#33689=DIRECTION('ref_axis',(1.,0.,0.));
#33690=DIRECTION('center_axis',(0.,0.,1.));
#33691=DIRECTION('ref_axis',(1.,0.,0.));
#33692=DIRECTION('',(0.,0.,1.));
#33693=DIRECTION('center_axis',(1.,0.,0.));
#33694=DIRECTION('ref_axis',(0.,1.,0.));
#33695=DIRECTION('',(0.,1.,0.));
#33696=DIRECTION('',(0.,1.,0.));
#33697=DIRECTION('',(0.,0.,1.));
#33698=DIRECTION('center_axis',(0.,0.,1.));
#33699=DIRECTION('ref_axis',(0.,-1.,0.));
#33700=DIRECTION('center_axis',(0.,0.,1.));
#33701=DIRECTION('ref_axis',(0.,-1.,0.));
#33702=DIRECTION('center_axis',(0.,0.,1.));
#33703=DIRECTION('ref_axis',(0.,-1.,0.));
#33704=DIRECTION('',(0.,0.,1.));
#33705=DIRECTION('center_axis',(0.,-1.,0.));
#33706=DIRECTION('ref_axis',(1.,0.,0.));
#33707=DIRECTION('',(1.,0.,0.));
#33708=DIRECTION('',(1.,0.,0.));
#33709=DIRECTION('',(0.,0.,1.));
#33710=DIRECTION('center_axis',(-0.707106781186547,-0.707106781186548,0.));
#33711=DIRECTION('ref_axis',(0.707106781186548,-0.707106781186547,0.));
#33712=DIRECTION('',(0.707106781186548,-0.707106781186547,0.));
#33713=DIRECTION('',(0.707106781186548,-0.707106781186547,0.));
#33714=DIRECTION('',(0.,0.,1.));
#33715=DIRECTION('center_axis',(-1.,0.,0.));
#33716=DIRECTION('ref_axis',(0.,-1.,0.));
#33717=DIRECTION('',(0.,-1.,0.));
#33718=DIRECTION('',(0.,-1.,0.));
#33719=DIRECTION('',(0.,0.,1.));
#33720=DIRECTION('center_axis',(0.,0.,1.));
#33721=DIRECTION('ref_axis',(1.,0.,0.));
#33722=DIRECTION('center_axis',(0.,0.,1.));
#33723=DIRECTION('ref_axis',(1.,0.,0.));
#33724=DIRECTION('center_axis',(0.,0.,-1.));
#33725=DIRECTION('ref_axis',(1.,0.,0.));
#33726=DIRECTION('',(0.,0.,1.));
#33727=DIRECTION('center_axis',(-0.46947156278589,-0.882947592858928,0.));
#33728=DIRECTION('ref_axis',(0.882947592858928,-0.46947156278589,0.));
#33729=DIRECTION('',(0.882947592858928,-0.46947156278589,0.));
#33730=DIRECTION('',(0.882947592858928,-0.46947156278589,0.));
#33731=DIRECTION('',(0.,0.,1.));
#33732=DIRECTION('center_axis',(0.,-1.,0.));
#33733=DIRECTION('ref_axis',(1.,0.,0.));
#33734=DIRECTION('',(1.,0.,0.));
#33735=DIRECTION('',(1.,0.,0.));
#33736=DIRECTION('',(0.,0.,1.));
#33737=DIRECTION('center_axis',(-1.,0.,0.));
#33738=DIRECTION('ref_axis',(0.,-1.,0.));
#33739=DIRECTION('',(0.,-1.,0.));
#33740=DIRECTION('',(0.,-1.,0.));
#33741=DIRECTION('center_axis',(0.,0.,1.));
#33742=DIRECTION('ref_axis',(1.,0.,0.));
#33743=DIRECTION('center_axis',(0.,0.,1.));
#33744=DIRECTION('ref_axis',(1.,0.,0.));
#33745=DIRECTION('',(0.,0.,1.));
#33746=DIRECTION('',(1.,0.,0.));
#33747=DIRECTION('',(0.,0.,1.));
#33748=DIRECTION('',(1.,0.,0.));
#124427=CARTESIAN_POINT('',(0.,0.,0.));
#125618=CARTESIAN_POINT('Origin',(0.000260570142325415,45.1297404501394,
36.));
#125619=CARTESIAN_POINT('',(0.00026057014232539,45.1297404501426,32.9999999993629));
#125620=CARTESIAN_POINT('',(0.00026057014232539,45.1297404501426,39.0000000006371));
#125621=CARTESIAN_POINT('Origin',(0.000260570142325415,45.1297404501395,
36.));
#125622=CARTESIAN_POINT('Origin',(0.000260570142325751,45.1297404501489,
36.));
#125623=CARTESIAN_POINT('',(0.000117784559150455,41.1297404526879,39.));
#125624=CARTESIAN_POINT('',(0.000260570142325048,45.1297404501394,39.));
#125625=CARTESIAN_POINT('Origin',(0.000117784559150088,41.1297404526879,
36.));
#125626=CARTESIAN_POINT('Origin',(0.000117784559149936,41.1297404526879,
36.));
#125627=CARTESIAN_POINT('Origin',(0.000260570142326236,45.1297404501394,
96.));
#125628=CARTESIAN_POINT('',(0.00026057014232539,45.1297404501426,92.9999999993629));
#125629=CARTESIAN_POINT('',(0.00026057014232539,45.1297404501426,99.0000000006371));
#125630=CARTESIAN_POINT('Origin',(0.000260570142326236,45.1297404501395,
96.));
#125631=CARTESIAN_POINT('Origin',(0.000260570142326572,45.1297404501489,
96.));
#125632=CARTESIAN_POINT('',(0.000117784559151277,41.1297404526879,99.));
#125633=CARTESIAN_POINT('',(0.000260570142325869,45.1297404501394,99.));
#125634=CARTESIAN_POINT('Origin',(0.000117784559150909,41.1297404526879,
96.));
#125635=CARTESIAN_POINT('Origin',(0.000117784559151046,41.1297404526879,
96.));
#125636=CARTESIAN_POINT('Origin',(7.20026057014233,45.1297404501395,26.));
#125637=CARTESIAN_POINT('',(0.000260570142325278,45.1297404501395,26.));
#125638=CARTESIAN_POINT('',(0.000260570142325278,45.1297404501395,106.));
#125639=CARTESIAN_POINT('',(0.000260570142325278,45.1297404501395,26.));
#125640=CARTESIAN_POINT('',(7.20026057014233,45.1297404501395,106.));
#125641=CARTESIAN_POINT('',(7.20026057014233,45.1297404501395,106.));
#125642=CARTESIAN_POINT('',(7.20026057014233,45.1297404501395,26.));
#125643=CARTESIAN_POINT('',(7.20026057014233,45.1297404501395,26.));
#125644=CARTESIAN_POINT('',(0.000260570142325278,45.1297404501395,26.));
#125645=CARTESIAN_POINT('',(7.20026057014233,45.1297404501395,26.));
#125646=CARTESIAN_POINT('',(0.000260570142325278,45.1297404501395,26.));
#125647=CARTESIAN_POINT('Origin',(16.0005712344353,40.3838853813626,46.));
#125648=CARTESIAN_POINT('',(16.0005576038968,40.0020390449739,43.0244003328805));
#125649=CARTESIAN_POINT('',(16.0005576038968,40.0020390449739,48.9755996671195));
#125650=CARTESIAN_POINT('',(16.0005576038968,40.0020390450537,36.));
#125651=CARTESIAN_POINT('Origin',(16.0005712344353,40.3838853813626,46.));
#125652=CARTESIAN_POINT('Origin',(-25.9994287388058,40.3853846300409,46.));
#125653=CARTESIAN_POINT('',(-16.000205842957,40.3850276938095,43.));
#125654=CARTESIAN_POINT('Origin',(-16.000205842957,40.3850276938095,46.));
#125655=CARTESIAN_POINT('',(-14.1509424007594,40.3849616818491,43.));
#125656=CARTESIAN_POINT('',(-25.9994287388058,40.3853846300409,43.));
#125657=CARTESIAN_POINT('',(-14.2001947782207,40.6949634400972,43.0160596520708));
#125658=CARTESIAN_POINT('Ctrl Pts',(-14.1509424007594,40.384961681931,43.));
#125659=CARTESIAN_POINT('Ctrl Pts',(-14.1842343067511,40.4870767337193,
43.0000000000056));
#125660=CARTESIAN_POINT('Ctrl Pts',(-14.2001983851187,40.5939196884095,
43.0055622696198));
#125661=CARTESIAN_POINT('Ctrl Pts',(-14.2001947782208,40.6949634400972,
43.0160596520708));
#125662=CARTESIAN_POINT('',(-14.200125669996,42.6309634388637,44.0111601371654));
#125663=CARTESIAN_POINT('Origin',(-14.2002058441038,40.3849634402947,46.));
#125664=CARTESIAN_POINT('',(-13.700107822116,43.1309455903466,44.7919089438291));
#125665=CARTESIAN_POINT('Ctrl Pts',(-13.700107822116,43.1309455903466,44.7919089438292));
#125666=CARTESIAN_POINT('Ctrl Pts',(-13.7287138176145,43.1309466114776,
44.7919089438292));
#125667=CARTESIAN_POINT('Ctrl Pts',(-13.7588198896061,43.1282901354821,
44.7858171356271));
#125668=CARTESIAN_POINT('Ctrl Pts',(-13.8150242028358,43.1184187630571,
44.7637668516514));
#125669=CARTESIAN_POINT('Ctrl Pts',(-13.8411536038327,43.1112169321056,
44.7478820248202));
#125670=CARTESIAN_POINT('Ctrl Pts',(-13.942146077159,43.0763467034421,44.6731422398802));
#125671=CARTESIAN_POINT('Ctrl Pts',(-14.0082080214715,43.0299667749565,
44.5814744645503));
#125672=CARTESIAN_POINT('Ctrl Pts',(-14.1423359864052,42.8958483854512,
44.3486366205185));
#125673=CARTESIAN_POINT('Ctrl Pts',(-14.2001209716938,42.7625818225232,
44.1597969859191));
#125674=CARTESIAN_POINT('Ctrl Pts',(-14.2001256699959,42.6309634388638,
44.0111601371654));
#125675=CARTESIAN_POINT('',(-12.8001078226894,43.1309134635892,44.7919089438291));
#125676=CARTESIAN_POINT('',(-25.9993307164994,43.1313846282914,44.7919089438291));
#125677=CARTESIAN_POINT('',(-12.8001078226894,43.1309134635892,47.2080910561709));
#125678=CARTESIAN_POINT('Ctrl Pts',(-12.8001078226893,43.1309134635892,
47.2080910561709));
#125679=CARTESIAN_POINT('Ctrl Pts',(-12.7874290218161,43.1309130110017,
47.2080910561709));
#125680=CARTESIAN_POINT('Ctrl Pts',(-12.7747450872089,43.1317310514822,
47.2062354373186));
#125681=CARTESIAN_POINT('Ctrl Pts',(-12.7501661862404,43.1348375455173,
47.199133868969));
#125682=CARTESIAN_POINT('Ctrl Pts',(-12.7382804382214,43.1371385398321,
47.193861533145));
#125683=CARTESIAN_POINT('Ctrl Pts',(-12.7046747516163,43.1455281504129,
47.1743800110828));
#125684=CARTESIAN_POINT('Ctrl Pts',(-12.6851453672407,43.1532658613644,
47.1561143770981));
#125685=CARTESIAN_POINT('Ctrl Pts',(-12.6471649980075,43.1716314784724,
47.111298056684));
#125686=CARTESIAN_POINT('Ctrl Pts',(-12.6264424973877,43.1855881094717,
47.0757741121274));
#125687=CARTESIAN_POINT('Ctrl Pts',(-12.5778499600881,43.224674918756,46.9705448594992));
#125688=CARTESIAN_POINT('Ctrl Pts',(-12.5550921166024,43.2558293923731,
46.8746617707269));
#125689=CARTESIAN_POINT('Ctrl Pts',(-12.5029059493652,43.3441575831397,
46.5522053662921));
#125690=CARTESIAN_POINT('Ctrl Pts',(-12.5036463989442,43.3849028811463,
46.2522550206409));
#125691=CARTESIAN_POINT('Ctrl Pts',(-12.5036463989442,43.3849028811463,
45.7477449793591));
#125692=CARTESIAN_POINT('Ctrl Pts',(-12.5029059493652,43.3441575831397,
45.4477946337079));
#125693=CARTESIAN_POINT('Ctrl Pts',(-12.5550921166024,43.2558293923731,
45.1253382292731));
#125694=CARTESIAN_POINT('Ctrl Pts',(-12.5778499600881,43.224674918756,45.0294551405009));
#125695=CARTESIAN_POINT('Ctrl Pts',(-12.6264424973877,43.1855881094717,
44.9242258878726));
#125696=CARTESIAN_POINT('Ctrl Pts',(-12.6471649980075,43.1716314784724,
44.888701943316));
#125697=CARTESIAN_POINT('Ctrl Pts',(-12.6851453672407,43.1532658613644,
44.8438856229019));
#125698=CARTESIAN_POINT('Ctrl Pts',(-12.7046747516163,43.1455281504129,
44.8256199889173));
#125699=CARTESIAN_POINT('Ctrl Pts',(-12.7382804382214,43.1371385398321,
44.806138466855));
#125700=CARTESIAN_POINT('Ctrl Pts',(-12.7501661862404,43.1348375455173,
44.800866131031));
#125701=CARTESIAN_POINT('Ctrl Pts',(-12.7747450872089,43.1317310514822,
44.7937645626814));
#125702=CARTESIAN_POINT('Ctrl Pts',(-12.7874290218161,43.1309130110017,
44.7919089438292));
#125703=CARTESIAN_POINT('Ctrl Pts',(-12.8001078226893,43.1309134635892,
44.7919089438292));
#125704=CARTESIAN_POINT('',(-13.700107822116,43.1309455903466,47.2080910561709));
#125705=CARTESIAN_POINT('',(-25.9993307164994,43.1313846282914,47.2080910561709));
#125706=CARTESIAN_POINT('',(-14.200125669996,42.6309634388637,47.9888398628346));
#125707=CARTESIAN_POINT('Ctrl Pts',(-14.2001256699959,42.6309634388638,
47.9888398628346));
#125708=CARTESIAN_POINT('Ctrl Pts',(-14.2001209716939,42.7625818225232,
47.8402030140809));
#125709=CARTESIAN_POINT('Ctrl Pts',(-14.1423359864052,42.8958483854512,
47.6513633794815));
#125710=CARTESIAN_POINT('Ctrl Pts',(-14.0082080214715,43.0299667749565,
47.4185255354497));
#125711=CARTESIAN_POINT('Ctrl Pts',(-13.942146077159,43.0763467034421,47.3268577601199));
#125712=CARTESIAN_POINT('Ctrl Pts',(-13.8411536038327,43.1112169321056,
47.2521179751798));
#125713=CARTESIAN_POINT('Ctrl Pts',(-13.8150242028358,43.1184187630571,
47.2362331483486));
#125714=CARTESIAN_POINT('Ctrl Pts',(-13.7588198896061,43.1282901354821,
47.2141828643729));
#125715=CARTESIAN_POINT('Ctrl Pts',(-13.7287138176144,43.1309466114776,
47.2080910561708));
#125716=CARTESIAN_POINT('Ctrl Pts',(-13.7001078221159,43.1309455903466,
47.2080910561708));
#125717=CARTESIAN_POINT('',(-14.2001947782207,40.6949634400972,48.9839403479292));
#125718=CARTESIAN_POINT('Origin',(-14.2002058441038,40.3849634402947,46.));
#125719=CARTESIAN_POINT('',(-13.9073268007583,39.9878462041285,48.9736015544009));
#125720=CARTESIAN_POINT('Ctrl Pts',(-13.9073268007584,39.9878462041285,
48.973601554401));
#125721=CARTESIAN_POINT('Ctrl Pts',(-13.9960100566734,40.076535791615,48.9854450979406));
#125722=CARTESIAN_POINT('Ctrl Pts',(-14.0730534099154,40.1890412751135,
48.9961344807684));
#125723=CARTESIAN_POINT('Ctrl Pts',(-14.1751560019799,40.435594122051,49.0021062582817));
#125724=CARTESIAN_POINT('Ctrl Pts',(-14.2001992511613,40.5696583440676,
48.9969582287394));
#125725=CARTESIAN_POINT('Ctrl Pts',(-14.2001947782208,40.6949634400972,
48.9839403479292));
#125726=CARTESIAN_POINT('',(-13.0856980517762,39.1661587946801,48.7412793024013));
#125727=CARTESIAN_POINT('Origin',(-14.3044194064105,40.3849671603434,46.));
#125728=CARTESIAN_POINT('',(-11.6715054007694,38.5803218750975,48.3965797735301));
#125729=CARTESIAN_POINT('Ctrl Pts',(-11.6715054007694,38.5803218750975,
48.3965797735301));
#125730=CARTESIAN_POINT('Ctrl Pts',(-11.9310804859103,38.5803311409929,
48.3965797735301));
#125731=CARTESIAN_POINT('Ctrl Pts',(-12.2008654839661,38.6335041042047,
48.4388004161354));
#125732=CARTESIAN_POINT('Ctrl Pts',(-12.6901619533851,38.8388876989633,
48.5738923324279));
#125733=CARTESIAN_POINT('Ctrl Pts',(-12.9106059326522,38.9910541747943,
48.6634310729608));
#125734=CARTESIAN_POINT('Ctrl Pts',(-13.0856980517762,39.1661587946801,
48.7412793024013));
#125735=CARTESIAN_POINT('',(-9.57050540210797,38.5802468769672,48.3965797735301));
#125736=CARTESIAN_POINT('',(-25.9994931547856,38.5808333326384,48.3965797735301));
#125737=CARTESIAN_POINT('',(-6.03491922226453,40.0445867642791,48.980661345019));
#125738=CARTESIAN_POINT('Ctrl Pts',(-6.03491922226454,40.0445867642791,
48.980661345019));
#125739=CARTESIAN_POINT('Ctrl Pts',(-6.46491979272285,39.6146168916673,
48.9316012220604));
#125740=CARTESIAN_POINT('Ctrl Pts',(-6.98352950944328,39.2568425175939,
48.7941482303742));
#125741=CARTESIAN_POINT('Ctrl Pts',(-8.18737580567769,38.7250267702563,
48.519101496493));
#125742=CARTESIAN_POINT('Ctrl Pts',(-8.88897256914252,38.5802225487005,
48.3965797735301));
#125743=CARTESIAN_POINT('Ctrl Pts',(-9.57050540210795,38.5802468769672,
48.3965797735301));
#125744=CARTESIAN_POINT('',(-4.31517414500253,41.7642090685172,48.6639647170471));
#125745=CARTESIAN_POINT('Origin',(-5.69482187817972,40.3846598287309,46.));
#125746=CARTESIAN_POINT('',(-4.88081081954212,43.1299146855279,47.2097174218851));
#125747=CARTESIAN_POINT('Ctrl Pts',(-4.88081081954212,43.1299146855279,
47.2097174218852));
#125748=CARTESIAN_POINT('Ctrl Pts',(-4.82482221472671,43.1299126869364,
47.2097174218852));
#125749=CARTESIAN_POINT('Ctrl Pts',(-4.77320031795728,43.1241916785181,
47.2228273668612));
#125750=CARTESIAN_POINT('Ctrl Pts',(-4.67621148812538,43.104869821818,47.2652368623581));
#125751=CARTESIAN_POINT('Ctrl Pts',(-4.63083615831866,43.0912259898174,
47.2944976062002));
#125752=CARTESIAN_POINT('Ctrl Pts',(-4.50299531310249,43.0409837535405,
47.3962229005734));
#125753=CARTESIAN_POINT('Ctrl Pts',(-4.42918588082232,42.9947395232464,
47.4819738279894));
#125754=CARTESIAN_POINT('Ctrl Pts',(-4.28473708613121,42.8747600616692,
47.6785381778342));
#125755=CARTESIAN_POINT('Ctrl Pts',(-4.21173521992966,42.7838888359608,
47.808410822416));
#125756=CARTESIAN_POINT('Ctrl Pts',(-4.10948896604543,42.5724250222423,
48.0592085197964));
#125757=CARTESIAN_POINT('Ctrl Pts',(-4.08083503287425,42.4515873535033,
48.1801672395615));
#125758=CARTESIAN_POINT('Ctrl Pts',(-4.08084269258332,42.2370080209205,
48.3629383226615));
#125759=CARTESIAN_POINT('Ctrl Pts',(-4.09805029004739,42.1312231898084,
48.4421976606013));
#125760=CARTESIAN_POINT('Ctrl Pts',(-4.17859647402362,41.9330114055893,
48.5720688356092));
#125761=CARTESIAN_POINT('Ctrl Pts',(-4.23902256544589,41.8403552115939,
48.6245291895113));
#125762=CARTESIAN_POINT('Ctrl Pts',(-4.31517414500251,41.7642090685172,
48.6639647170472));
#125763=CARTESIAN_POINT('',(-7.19981081806464,43.1299974654728,47.209717421885));
#125764=CARTESIAN_POINT('',(-25.9993307420611,43.1306685406019,47.2097174218847));
#125765=CARTESIAN_POINT('',(-7.19981081806464,43.1299974654728,44.790282578115));
#125766=CARTESIAN_POINT('Ctrl Pts',(-7.19981081806464,43.1299974654728,
44.790282578115));
#125767=CARTESIAN_POINT('Ctrl Pts',(-7.21250680486427,43.1299979186738,
44.790282578115));
#125768=CARTESIAN_POINT('Ctrl Pts',(-7.22520787530932,43.1308190809083,
44.7921402324464));
#125769=CARTESIAN_POINT('Ctrl Pts',(-7.24981968793656,43.1339357989149,
44.7992497365215));
#125770=CARTESIAN_POINT('Ctrl Pts',(-7.26172119707253,43.13624393064,44.8045280031557));
#125771=CARTESIAN_POINT('Ctrl Pts',(-7.29537069273696,43.1446590481209,
44.8240319462818));
#125772=CARTESIAN_POINT('Ctrl Pts',(-7.31492435500479,43.1524197100444,
44.8423192550511));
#125773=CARTESIAN_POINT('Ctrl Pts',(-7.35294574461562,43.1708382902919,
44.8871870557474));
#125774=CARTESIAN_POINT('Ctrl Pts',(-7.37368596111585,43.1848338692446,
44.9227502546591));
#125775=CARTESIAN_POINT('Ctrl Pts',(-7.42230928437433,43.2240280671579,
45.0280938938583));
#125776=CARTESIAN_POINT('Ctrl Pts',(-7.44506219926235,43.2552667477377,
45.1240810706962));
#125777=CARTESIAN_POINT('Ctrl Pts',(-7.49721225591251,43.34385822923,45.4469741746507));
#125778=CARTESIAN_POINT('Ctrl Pts',(-7.49636431121142,43.3847241392164,
45.7473663615792));
#125779=CARTESIAN_POINT('Ctrl Pts',(-7.49636431121142,43.3847241392164,
46.2526336384208));
#125780=CARTESIAN_POINT('Ctrl Pts',(-7.49721225591251,43.34385822923,46.5530258253493));
#125781=CARTESIAN_POINT('Ctrl Pts',(-7.44506219926235,43.2552667477377,
46.8759189293038));
#125782=CARTESIAN_POINT('Ctrl Pts',(-7.42230928437433,43.2240280671579,
46.9719061061417));
#125783=CARTESIAN_POINT('Ctrl Pts',(-7.37368596111585,43.1848338692446,
47.0772497453409));
#125784=CARTESIAN_POINT('Ctrl Pts',(-7.35294574461562,43.1708382902919,
47.1128129442526));
#125785=CARTESIAN_POINT('Ctrl Pts',(-7.31492435500479,43.1524197100444,
47.1576807449489));
#125786=CARTESIAN_POINT('Ctrl Pts',(-7.29537069273696,43.1446590481209,
47.1759680537182));
#125787=CARTESIAN_POINT('Ctrl Pts',(-7.26172119707253,43.13624393064,47.1954719968443));
#125788=CARTESIAN_POINT('Ctrl Pts',(-7.24981968793656,43.1339357989149,
47.2007502634786));
#125789=CARTESIAN_POINT('Ctrl Pts',(-7.22520787530932,43.1308190809083,
47.2078597675536));
#125790=CARTESIAN_POINT('Ctrl Pts',(-7.21250680486427,43.1299979186738,
47.209717421885));
#125791=CARTESIAN_POINT('Ctrl Pts',(-7.19981081806464,43.1299974654728,
47.209717421885));
#125792=CARTESIAN_POINT('',(-4.88081081954212,43.1299146855279,44.7902825781149));
#125793=CARTESIAN_POINT('',(-25.9993307420611,43.1306685406019,44.7902825781153));
#125794=CARTESIAN_POINT('',(-4.31517414500253,41.7642090685172,43.3360352829528));
#125795=CARTESIAN_POINT('Ctrl Pts',(-4.31517414500254,41.7642090685172,
43.3360352829528));
#125796=CARTESIAN_POINT('Ctrl Pts',(-4.2390225654459,41.8403552115938,43.3754708104887));
#125797=CARTESIAN_POINT('Ctrl Pts',(-4.17859647402362,41.9330114055893,
43.4279311643908));
#125798=CARTESIAN_POINT('Ctrl Pts',(-4.09805029004739,42.1312231898084,
43.5578023393987));
#125799=CARTESIAN_POINT('Ctrl Pts',(-4.08084269258332,42.2370080209205,
43.6370616773385));
#125800=CARTESIAN_POINT('Ctrl Pts',(-4.08083503287425,42.4515873535033,
43.8198327604385));
#125801=CARTESIAN_POINT('Ctrl Pts',(-4.10948896604543,42.5724250222423,
43.9407914802036));
#125802=CARTESIAN_POINT('Ctrl Pts',(-4.21173521992966,42.7838888359608,
44.191589177584));
#125803=CARTESIAN_POINT('Ctrl Pts',(-4.28473708613121,42.8747600616692,
44.3214618221658));
#125804=CARTESIAN_POINT('Ctrl Pts',(-4.42918588082232,42.9947395232464,
44.5180261720106));
#125805=CARTESIAN_POINT('Ctrl Pts',(-4.50299531310249,43.0409837535405,
44.6037770994266));
#125806=CARTESIAN_POINT('Ctrl Pts',(-4.63083615831866,43.0912259898174,
44.7055023937998));
#125807=CARTESIAN_POINT('Ctrl Pts',(-4.67621148812537,43.104869821818,44.7347631376419));
#125808=CARTESIAN_POINT('Ctrl Pts',(-4.77320031795728,43.1241916785181,
44.7771726331388));
#125809=CARTESIAN_POINT('Ctrl Pts',(-4.82482221472671,43.1299126869364,
44.7902825781148));
#125810=CARTESIAN_POINT('Ctrl Pts',(-4.88081081954212,43.1299146855279,
44.7902825781148));
#125811=CARTESIAN_POINT('',(-5.69482187817968,40.384659828731,43.));
#125812=CARTESIAN_POINT('Origin',(-5.69482187817972,40.3846598287309,46.));
#125813=CARTESIAN_POINT('',(5.69537693071232,40.384253239671,43.));
#125814=CARTESIAN_POINT('',(-25.9994287388058,40.3853846300409,43.));
#125815=CARTESIAN_POINT('',(4.3155751451931,41.7640550251902,43.3361150636597));
#125816=CARTESIAN_POINT('Origin',(5.69537693071237,40.3842532396709,46.));
#125817=CARTESIAN_POINT('',(4.88126057014233,43.1297404501394,44.7906780580687));
#125818=CARTESIAN_POINT('Ctrl Pts',(4.88126057014233,43.1297404501394,44.7906780580686));
#125819=CARTESIAN_POINT('Ctrl Pts',(4.82527855129633,43.1297404501394,44.7906735213083));
#125820=CARTESIAN_POINT('Ctrl Pts',(4.77366641546815,43.1240229215084,44.7775580917314));
#125821=CARTESIAN_POINT('Ctrl Pts',(4.6766881693441,43.1047100794269,44.7351374178226));
#125822=CARTESIAN_POINT('Ctrl Pts',(4.63131473335929,43.0910704365374,44.7058682945448));
#125823=CARTESIAN_POINT('Ctrl Pts',(4.50347730469684,43.040841140764,44.6041166977585));
#125824=CARTESIAN_POINT('Ctrl Pts',(4.42966809762419,42.9946063244288,44.5183478507339));
#125825=CARTESIAN_POINT('Ctrl Pts',(4.28521059479939,42.8746430433406,44.3217402796909));
#125826=CARTESIAN_POINT('Ctrl Pts',(4.21219885970608,42.7837779689826,44.1918390912013));
#125827=CARTESIAN_POINT('Ctrl Pts',(4.10993073305515,42.5723177386494,43.9409875062198));
#125828=CARTESIAN_POINT('Ctrl Pts',(4.08126491520575,42.4514774729932,43.8200033709792));
#125829=CARTESIAN_POINT('Ctrl Pts',(4.08125725528774,42.2368922872938,43.6371990515189));
#125830=CARTESIAN_POINT('Ctrl Pts',(4.09845674449903,42.1311064778841,43.5579277928478));
#125831=CARTESIAN_POINT('Ctrl Pts',(4.17899207419104,41.9328803074183,43.4280312090116));
#125832=CARTESIAN_POINT('Ctrl Pts',(4.23941854432906,41.8402116260542,43.375558776258));
#125833=CARTESIAN_POINT('Ctrl Pts',(4.31557514519307,41.7640550251902,43.3361150636597));
#125834=CARTESIAN_POINT('',(7.20026057014233,43.1297404501395,44.7908660063353));
#125835=CARTESIAN_POINT('',(6.04076057014233,43.1297404501395,44.790772032202));
#125836=CARTESIAN_POINT('',(7.20026057014233,43.1297404501395,47.2091339936647));
#125837=CARTESIAN_POINT('Ctrl Pts',(7.20026057014233,43.1297404501395,47.2091339936647));
#125838=CARTESIAN_POINT('Ctrl Pts',(7.21294682501949,43.1297404501395,47.2091329653848));
#125839=CARTESIAN_POINT('Ctrl Pts',(7.22563810372133,43.1305598955788,47.2072760701667));
#125840=CARTESIAN_POINT('Ctrl Pts',(7.25023479260245,43.1336713801016,47.2001704115751));
#125841=CARTESIAN_POINT('Ctrl Pts',(7.26213075345329,43.1359764055222,47.1948942718855));
#125842=CARTESIAN_POINT('Ctrl Pts',(7.29576491915057,43.144380828481,47.1753983698309));
#125843=CARTESIAN_POINT('Ctrl Pts',(7.31531022822448,43.152132358212,47.1571188348341));
#125844=CARTESIAN_POINT('Ctrl Pts',(7.35331775020092,43.1705301900497,47.1122694969576));
#125845=CARTESIAN_POINT('Ctrl Pts',(7.3740522567382,43.1845108420159,47.0767203752737));
#125846=CARTESIAN_POINT('Ctrl Pts',(7.4226663467744,43.2236642757062,46.9714177547315));
#125847=CARTESIAN_POINT('Ctrl Pts',(7.44542247694709,43.2548716957552,46.8754679026737));
#125848=CARTESIAN_POINT('Ctrl Pts',(7.49758960390303,43.3433662832606,46.5527314566462));
#125849=CARTESIAN_POINT('Ctrl Pts',(7.49678217092917,43.3841889379055,46.2524977920887));
#125850=CARTESIAN_POINT('Ctrl Pts',(7.49678217092917,43.3841889379055,45.7475022079113));
#125851=CARTESIAN_POINT('Ctrl Pts',(7.49758960390303,43.3433662832606,45.4472685433538));
#125852=CARTESIAN_POINT('Ctrl Pts',(7.44542247694709,43.2548716957552,45.1245320973263));
#125853=CARTESIAN_POINT('Ctrl Pts',(7.4226663467744,43.2236642757062,45.0285822452685));
#125854=CARTESIAN_POINT('Ctrl Pts',(7.3740522567382,43.1845108420159,44.9232796247263));
#125855=CARTESIAN_POINT('Ctrl Pts',(7.35331775020092,43.1705301900497,44.8877305030425));
#125856=CARTESIAN_POINT('Ctrl Pts',(7.31531022822448,43.152132358212,44.8428811651659));
#125857=CARTESIAN_POINT('Ctrl Pts',(7.29576491915057,43.144380828481,44.8246016301691));
#125858=CARTESIAN_POINT('Ctrl Pts',(7.26213075345329,43.1359764055222,44.8051057281145));
#125859=CARTESIAN_POINT('Ctrl Pts',(7.25023479260246,43.1336713801016,44.7998295884249));
#125860=CARTESIAN_POINT('Ctrl Pts',(7.22563810372133,43.1305598955788,44.7927239298333));
#125861=CARTESIAN_POINT('Ctrl Pts',(7.2129468250195,43.1297404501395,44.7908670346152));
#125862=CARTESIAN_POINT('Ctrl Pts',(7.20026057014233,43.1297404501395,44.7908660063354));
#125863=CARTESIAN_POINT('',(4.88126057014233,43.1297404501394,47.2093219419313));
#125864=CARTESIAN_POINT('',(6.04076057014233,43.1297404501395,47.209227967798));
#125865=CARTESIAN_POINT('',(4.3155751451931,41.7640550251902,48.6638849363403));
#125866=CARTESIAN_POINT('Ctrl Pts',(4.31557514519307,41.7640550251902,48.6638849363403));
#125867=CARTESIAN_POINT('Ctrl Pts',(4.23941854432905,41.8402116260542,48.624441223742));
#125868=CARTESIAN_POINT('Ctrl Pts',(4.17899207419104,41.9328803074183,48.5719687909884));
#125869=CARTESIAN_POINT('Ctrl Pts',(4.09845674449903,42.1311064778841,48.4420722071522));
#125870=CARTESIAN_POINT('Ctrl Pts',(4.08125725528774,42.2368922872938,48.3628009484811));
#125871=CARTESIAN_POINT('Ctrl Pts',(4.08126491520575,42.4514774729932,48.1799966290209));
#125872=CARTESIAN_POINT('Ctrl Pts',(4.10993073305514,42.5723177386493,48.0590124937802));
#125873=CARTESIAN_POINT('Ctrl Pts',(4.21219885970608,42.7837779689826,47.8081609087987));
#125874=CARTESIAN_POINT('Ctrl Pts',(4.28521059479939,42.8746430433406,47.6782597203091));
#125875=CARTESIAN_POINT('Ctrl Pts',(4.42966809762419,42.9946063244288,47.4816521492661));
#125876=CARTESIAN_POINT('Ctrl Pts',(4.50347730469684,43.040841140764,47.3958833022415));
#125877=CARTESIAN_POINT('Ctrl Pts',(4.63131473335929,43.0910704365374,47.2941317054552));
#125878=CARTESIAN_POINT('Ctrl Pts',(4.6766881693441,43.1047100794269,47.2648625821774));
#125879=CARTESIAN_POINT('Ctrl Pts',(4.77366641546815,43.1240229215084,47.2224419082686));
#125880=CARTESIAN_POINT('Ctrl Pts',(4.82527855129632,43.1297404501394,47.2093264786917));
#125881=CARTESIAN_POINT('Ctrl Pts',(4.88126057014233,43.1297404501394,47.2093219419314));
#125882=CARTESIAN_POINT('',(6.03525883703878,40.0443713333445,48.9806859172054));
#125883=CARTESIAN_POINT('Origin',(5.69537693071237,40.3842532396709,46.));
#125884=CARTESIAN_POINT('',(9.57079274297153,38.5799052392773,48.3968369781132));
#125885=CARTESIAN_POINT('Ctrl Pts',(9.57079274297153,38.5799052392773,48.3968369781133));
#125886=CARTESIAN_POINT('Ctrl Pts',(9.5707332488234,38.5799052392773,48.3968369765146));
#125887=CARTESIAN_POINT('Ctrl Pts',(9.5706737548282,38.5799052403392,48.3968369757153));
#125888=CARTESIAN_POINT('Ctrl Pts',(8.88909486927775,38.5799295702497,48.3968369757153));
#125889=CARTESIAN_POINT('Ctrl Pts',(8.1875100639932,38.724779883745,48.519320896401));
#125890=CARTESIAN_POINT('Ctrl Pts',(6.98374971135328,39.2566553618154,48.7942694455703));
#125891=CARTESIAN_POINT('Ctrl Pts',(6.4652044862175,39.6144256841659,48.9316635383853));
#125892=CARTESIAN_POINT('Ctrl Pts',(6.03525883703881,40.0443713333445,48.9806859172054));
#125893=CARTESIAN_POINT('',(11.6717927429715,38.5799052392773,48.3968934308243));
#125894=CARTESIAN_POINT('',(10.6212927429715,38.5799052392773,48.3968652044688));
#125895=CARTESIAN_POINT('',(13.0860063053446,39.1656916769042,48.7414869339534));
#125896=CARTESIAN_POINT('Ctrl Pts',(13.0860063053446,39.1656916769042,48.7414869339534));
#125897=CARTESIAN_POINT('Ctrl Pts',(12.9115776150688,38.9912629866284,48.663969269128));
#125898=CARTESIAN_POINT('Ctrl Pts',(12.6925492447761,38.8399015743528,48.5750351340623));
#125899=CARTESIAN_POINT('Ctrl Pts',(12.2039210685268,38.6336428861301,48.4395838913209));
#125900=CARTESIAN_POINT('Ctrl Pts',(11.9328135534399,38.5799052392773,48.3969004440812));
#125901=CARTESIAN_POINT('Ctrl Pts',(11.6717927429715,38.5799052392773,48.3968934308244));
#125902=CARTESIAN_POINT('',(13.9076643850834,39.987349756643,48.973667809827));
#125903=CARTESIAN_POINT('Origin',(14.3042605619825,40.383945933542,46.));
#125904=CARTESIAN_POINT('',(14.2005576038968,40.6944565378947,48.9838876432241));
#125905=CARTESIAN_POINT('Ctrl Pts',(14.2005576038968,40.6944565378295,48.9838876425972));
#125906=CARTESIAN_POINT('Ctrl Pts',(14.2005576038968,40.6944446389709,48.9838888808066));
#125907=CARTESIAN_POINT('Ctrl Pts',(14.2005576036844,40.6944327401719,48.9838901189378));
#125908=CARTESIAN_POINT('Ctrl Pts',(14.2005531444961,40.5695128967916,48.996887916041));
#125909=CARTESIAN_POINT('Ctrl Pts',(14.1756575752172,40.4358460629751,49.0020722846323));
#125910=CARTESIAN_POINT('Ctrl Pts',(14.0741268986634,40.1899012740497,48.9962434199587));
#125911=CARTESIAN_POINT('Ctrl Pts',(13.9975074091711,40.0776069665203,48.9856559212044));
#125912=CARTESIAN_POINT('Ctrl Pts',(13.9087580506029,39.988444692808,48.9738136974118));
#125913=CARTESIAN_POINT('Ctrl Pts',(13.9082116449317,39.9878970164913,48.9737408027343));
#125914=CARTESIAN_POINT('Ctrl Pts',(13.9076643850834,39.987349756643,48.973667809827));
#125915=CARTESIAN_POINT('',(14.2005576038968,42.6304565378295,47.9882672716729));
#125916=CARTESIAN_POINT('Origin',(14.2005576038968,40.383949635364,46.));
#125917=CARTESIAN_POINT('',(13.7005576038968,43.1304565378295,47.2069788251679));
#125918=CARTESIAN_POINT('Ctrl Pts',(13.7005576038968,43.1304565378295,47.206978825168));
#125919=CARTESIAN_POINT('Ctrl Pts',(13.7005635533611,43.1304565378295,47.2069788246847));
#125920=CARTESIAN_POINT('Ctrl Pts',(13.7005695027606,43.1304565377233,47.2069788244431));
#125921=CARTESIAN_POINT('Ctrl Pts',(13.7349434333177,43.1304553106978,47.2069788244431));
#125922=CARTESIAN_POINT('Ctrl Pts',(13.7667215268191,43.1269938687308,47.2149030662356));
#125923=CARTESIAN_POINT('Ctrl Pts',(13.8263020113281,43.1153320791706,47.240899990775));
#125924=CARTESIAN_POINT('Ctrl Pts',(13.8540993385831,43.1071092325231,47.2589741809338));
#125925=CARTESIAN_POINT('Ctrl Pts',(13.9319395673727,43.0771707831725,47.3224216534088));
#125926=CARTESIAN_POINT('Ctrl Pts',(13.9761986813102,43.0500508066361,47.3767434803275));
#125927=CARTESIAN_POINT('Ctrl Pts',(14.070024541769,42.9755247782782,47.5143570677025));
#125928=CARTESIAN_POINT('Ctrl Pts',(14.1174300227276,42.916521123884,47.6124763023577));
#125929=CARTESIAN_POINT('Ctrl Pts',(14.1829744042219,42.7817463851036,47.8068079086529));
#125930=CARTESIAN_POINT('Ctrl Pts',(14.2005576038968,42.7058286960662,47.9031056458044));
#125931=CARTESIAN_POINT('Ctrl Pts',(14.2005576038968,42.6304565378295,47.9882672716729));
#125932=CARTESIAN_POINT('',(12.8005576038968,43.1304565378295,47.2070519271956));
#125933=CARTESIAN_POINT('',(13.2505576038968,43.1304565378295,47.2070153761818));
#125934=CARTESIAN_POINT('',(12.8005576038968,43.1304565378295,44.7929480728044));
#125935=CARTESIAN_POINT('Ctrl Pts',(12.8005576038968,43.1304565378295,44.7929480728044));
#125936=CARTESIAN_POINT('Ctrl Pts',(12.8005540342567,43.1304565378295,44.7929480725144));
#125937=CARTESIAN_POINT('Ctrl Pts',(12.800550464617,43.1304565378932,44.7929480723695));
#125938=CARTESIAN_POINT('Ctrl Pts',(12.8005468949777,43.1304565380206,44.7929480723695));
#125939=CARTESIAN_POINT('Ctrl Pts',(12.7878790745653,43.1304569902162,44.7929480723695));
#125940=CARTESIAN_POINT('Ctrl Pts',(12.775206184161,43.1312745218071,44.7948023896052));
#125941=CARTESIAN_POINT('Ctrl Pts',(12.7506486750991,43.1343773655443,44.801898883713));
#125942=CARTESIAN_POINT('Ctrl Pts',(12.738773266856,43.1366751949132,44.8071674273607));
#125943=CARTESIAN_POINT('Ctrl Pts',(12.7051965550664,43.1450524580709,44.826634614644));
#125944=CARTESIAN_POINT('Ctrl Pts',(12.6856835914487,43.1527778071505,44.8448863925531));
#125945=CARTESIAN_POINT('Ctrl Pts',(12.6477316006356,43.1711140657731,44.8896697992274));
#125946=CARTESIAN_POINT('Ctrl Pts',(12.6270220730305,43.1850482619964,44.9251686425469));
#125947=CARTESIAN_POINT('Ctrl Pts',(12.5784538537086,43.2240722091775,45.0303247407441));
#125948=CARTESIAN_POINT('Ctrl Pts',(12.5556965844494,43.2551755942419,45.126141257432));
#125949=CARTESIAN_POINT('Ctrl Pts',(12.5034979555493,43.3433419209884,45.4483186441275));
#125950=CARTESIAN_POINT('Ctrl Pts',(12.5041748497398,43.3840101920279,45.7479867774995));
#125951=CARTESIAN_POINT('Ctrl Pts',(12.5041748497398,43.3840101920279,46.2520132225005));
#125952=CARTESIAN_POINT('Ctrl Pts',(12.5034979555493,43.3433419209884,46.5516813558725));
#125953=CARTESIAN_POINT('Ctrl Pts',(12.5556965844494,43.2551755942419,46.873858742568));
#125954=CARTESIAN_POINT('Ctrl Pts',(12.5784538537086,43.2240722091775,46.9696752592559));
#125955=CARTESIAN_POINT('Ctrl Pts',(12.6270220730305,43.1850482619964,47.0748313574531));
#125956=CARTESIAN_POINT('Ctrl Pts',(12.6477316006356,43.1711140657731,47.1103302007727));
#125957=CARTESIAN_POINT('Ctrl Pts',(12.6856835914487,43.1527778071505,47.1551136074469));
#125958=CARTESIAN_POINT('Ctrl Pts',(12.7051965550664,43.1450524580709,47.173365385356));
#125959=CARTESIAN_POINT('Ctrl Pts',(12.738773266856,43.1366751949132,47.1928325726393));
#125960=CARTESIAN_POINT('Ctrl Pts',(12.7506486750991,43.1343773655443,47.198101116287));
#125961=CARTESIAN_POINT('Ctrl Pts',(12.775206184161,43.1312745218071,47.2051976103948));
#125962=CARTESIAN_POINT('Ctrl Pts',(12.7878790745653,43.1304569902162,47.2070519276305));
#125963=CARTESIAN_POINT('Ctrl Pts',(12.800550464617,43.1304565378932,47.2070519276305));
#125964=CARTESIAN_POINT('Ctrl Pts',(12.8005540342567,43.1304565378295,47.2070519274856));
#125965=CARTESIAN_POINT('Ctrl Pts',(12.8005576038968,43.1304565378295,47.2070519271956));
#125966=CARTESIAN_POINT('',(13.7005576038968,43.1304565378295,44.7930211748321));
#125967=CARTESIAN_POINT('',(13.2505576038968,43.1304565378295,44.7929846238182));
#125968=CARTESIAN_POINT('',(14.2005576038968,42.6304565378295,44.0117327283271));
#125969=CARTESIAN_POINT('Ctrl Pts',(14.2005576038968,42.6304565378295,44.0117327283271));
#125970=CARTESIAN_POINT('Ctrl Pts',(14.2005576038968,42.7058286960662,44.0968943541956));
#125971=CARTESIAN_POINT('Ctrl Pts',(14.1829744042219,42.7817463851036,44.1931920913471));
#125972=CARTESIAN_POINT('Ctrl Pts',(14.1174300227276,42.916521123884,44.3875236976423));
#125973=CARTESIAN_POINT('Ctrl Pts',(14.070024541769,42.9755247782782,44.4856429322975));
#125974=CARTESIAN_POINT('Ctrl Pts',(13.9761986813102,43.0500508066361,44.6232565196725));
#125975=CARTESIAN_POINT('Ctrl Pts',(13.9319395673727,43.0771707831725,44.6775783465912));
#125976=CARTESIAN_POINT('Ctrl Pts',(13.8540993385831,43.1071092325231,44.7410258190662));
#125977=CARTESIAN_POINT('Ctrl Pts',(13.8263020113281,43.1153320791706,44.759100009225));
#125978=CARTESIAN_POINT('Ctrl Pts',(13.7667215268191,43.1269938687308,44.7850969337644));
#125979=CARTESIAN_POINT('Ctrl Pts',(13.7349434333177,43.1304553106978,44.7930211755569));
#125980=CARTESIAN_POINT('Ctrl Pts',(13.7005695027606,43.1304565377233,44.7930211755569));
#125981=CARTESIAN_POINT('Ctrl Pts',(13.7005635533611,43.1304565378295,44.7930211753153));
#125982=CARTESIAN_POINT('Ctrl Pts',(13.7005576038968,43.1304565378295,44.793021174832));
#125983=CARTESIAN_POINT('',(14.2005576038968,40.6944565378947,43.0161123567759));
#125984=CARTESIAN_POINT('Origin',(14.2005576038968,40.383949635364,46.));
#125985=CARTESIAN_POINT('',(14.1511293052103,40.3839513998532,43.));
#125986=CARTESIAN_POINT('Ctrl Pts',(14.1511293052103,40.3839513999301,43.));
#125987=CARTESIAN_POINT('Ctrl Pts',(14.184533612433,40.4862144071147,43.0000000000053));
#125988=CARTESIAN_POINT('Ctrl Pts',(14.2005539915515,40.5932423327881,43.0055811103851));
#125989=CARTESIAN_POINT('Ctrl Pts',(14.2005576036844,40.6944327401719,43.0161098810622));
#125990=CARTESIAN_POINT('Ctrl Pts',(14.2005576038968,40.6944446389709,43.0161111191934));
#125991=CARTESIAN_POINT('Ctrl Pts',(14.2005576038968,40.6944565378295,43.0161123574028));
#125992=CARTESIAN_POINT('',(16.0005576038968,40.3838853818492,42.9999999980887));
#125993=CARTESIAN_POINT('',(-25.9994287388058,40.3853846300409,43.));
#125994=CARTESIAN_POINT('Origin',(16.0005576038968,40.3838853818492,46.));
#125995=CARTESIAN_POINT('Origin',(16.0005576038968,40.3838853818492,46.));
#125996=CARTESIAN_POINT('',(13.9076643850834,39.987349756643,43.026332190173));
#125997=CARTESIAN_POINT('Ctrl Pts',(13.9076643850834,39.987349756643,43.026332190173));
#125998=CARTESIAN_POINT('Ctrl Pts',(13.9082116449317,39.9878970164913,43.0262591972657));
#125999=CARTESIAN_POINT('Ctrl Pts',(13.9087580506029,39.988444692808,43.0261863025882));
#126000=CARTESIAN_POINT('Ctrl Pts',(13.9975074091711,40.0776069665203,43.0143440787957));
#126001=CARTESIAN_POINT('Ctrl Pts',(14.0741268986634,40.1899012740497,43.0037565800413));
#126002=CARTESIAN_POINT('Ctrl Pts',(14.1345364020809,40.3362353976012,43.0002884772731));
#126003=CARTESIAN_POINT('Ctrl Pts',(14.1432949797111,40.3599676160584,42.9999999999988));
#126004=CARTESIAN_POINT('Ctrl Pts',(14.1511293052103,40.3839513999301,43.));
#126005=CARTESIAN_POINT('',(13.0860063053446,39.1656916769042,43.2585130660466));
#126006=CARTESIAN_POINT('Origin',(14.3042605619825,40.383945933542,46.));
#126007=CARTESIAN_POINT('',(11.6717927429715,38.5799052392773,43.6031065691757));
#126008=CARTESIAN_POINT('Ctrl Pts',(11.6717927429715,38.5799052392773,43.6031065691757));
#126009=CARTESIAN_POINT('Ctrl Pts',(11.9328135534399,38.5799052392773,43.6030995559188));
#126010=CARTESIAN_POINT('Ctrl Pts',(12.2039210685268,38.6336428861301,43.5604161086791));
#126011=CARTESIAN_POINT('Ctrl Pts',(12.6925492447761,38.8399015743528,43.4249648659377));
#126012=CARTESIAN_POINT('Ctrl Pts',(12.9115776150688,38.9912629866284,43.3360307308721));
#126013=CARTESIAN_POINT('Ctrl Pts',(13.0860063053446,39.1656916769042,43.2585130660466));
#126014=CARTESIAN_POINT('',(9.57079274297153,38.5799052392773,43.6031630218867));
#126015=CARTESIAN_POINT('',(10.6212927429715,38.5799052392773,43.6031347955312));
#126016=CARTESIAN_POINT('',(6.03525883703878,40.0443713333445,43.0193140827946));
#126017=CARTESIAN_POINT('Ctrl Pts',(6.03525883703881,40.0443713333445,43.0193140827946));
#126018=CARTESIAN_POINT('Ctrl Pts',(6.4652044862175,39.6144256841659,43.0683364616148));
#126019=CARTESIAN_POINT('Ctrl Pts',(6.98374971135328,39.2566553618154,43.2057305544297));
#126020=CARTESIAN_POINT('Ctrl Pts',(8.1875100639932,38.724779883745,43.480679103599));
#126021=CARTESIAN_POINT('Ctrl Pts',(8.88909486927775,38.5799295702497,43.6031630242847));
#126022=CARTESIAN_POINT('Ctrl Pts',(9.570614260986,38.5799052424629,43.6031630242847));
#126023=CARTESIAN_POINT('Ctrl Pts',(9.5706737548282,38.5799052403392,43.6031630242847));
#126024=CARTESIAN_POINT('Ctrl Pts',(9.5707332488234,38.5799052392773,43.6031630234854));
#126025=CARTESIAN_POINT('Ctrl Pts',(9.57079274297153,38.5799052392773,43.6031630218867));
#126026=CARTESIAN_POINT('Origin',(5.69537693071237,40.3842532396709,46.));
#126027=CARTESIAN_POINT('',(-6.03491922226453,40.0445867642791,43.019338654981));
#126028=CARTESIAN_POINT('Origin',(-5.69482187817972,40.3846598287309,46.));
#126029=CARTESIAN_POINT('',(-9.57050540210797,38.5802468769672,43.6034202264699));
#126030=CARTESIAN_POINT('Ctrl Pts',(-9.57050540210795,38.5802468769672,
43.60342022647));
#126031=CARTESIAN_POINT('Ctrl Pts',(-8.88897256914252,38.5802225487005,
43.60342022647));
#126032=CARTESIAN_POINT('Ctrl Pts',(-8.18737580567769,38.7250267702563,
43.480898503507));
#126033=CARTESIAN_POINT('Ctrl Pts',(-6.98352950944328,39.2568425175939,
43.2058517696258));
#126034=CARTESIAN_POINT('Ctrl Pts',(-6.46491979272286,39.6146168916673,
43.0683987779396));
#126035=CARTESIAN_POINT('Ctrl Pts',(-6.03491922226454,40.0445867642791,
43.019338654981));
#126036=CARTESIAN_POINT('',(-11.6715054007694,38.5803218750975,43.6034202264699));
#126037=CARTESIAN_POINT('',(-25.9994931547856,38.5808333326384,43.6034202264699));
#126038=CARTESIAN_POINT('',(-13.0856980517762,39.1661587946801,43.2587206975987));
#126039=CARTESIAN_POINT('Ctrl Pts',(-13.0856980517762,39.1661587946801,
43.2587206975987));
#126040=CARTESIAN_POINT('Ctrl Pts',(-12.9106059326522,38.9910541747943,
43.3365689270393));
#126041=CARTESIAN_POINT('Ctrl Pts',(-12.6901619533851,38.8388876989633,
43.4261076675721));
#126042=CARTESIAN_POINT('Ctrl Pts',(-12.2008654839661,38.6335041042048,
43.5611995838646));
#126043=CARTESIAN_POINT('Ctrl Pts',(-11.9310804859103,38.5803311409929,
43.6034202264699));
#126044=CARTESIAN_POINT('Ctrl Pts',(-11.6715054007694,38.5803218750975,
43.6034202264699));
#126045=CARTESIAN_POINT('',(-13.9073268007583,39.9878462041285,43.0263984455991));
#126046=CARTESIAN_POINT('Origin',(-14.3044194064105,40.3849671603434,46.));
#126047=CARTESIAN_POINT('Ctrl Pts',(-13.9073268007584,39.9878462041285,
43.0263984455991));
#126048=CARTESIAN_POINT('Ctrl Pts',(-13.9960100566734,40.076535791615,43.0145549020595));
#126049=CARTESIAN_POINT('Ctrl Pts',(-14.0730534099154,40.1890412751135,
43.0038655192316));
#126050=CARTESIAN_POINT('Ctrl Pts',(-14.1339891648514,40.3361862550399,
43.0003015081353));
#126051=CARTESIAN_POINT('Ctrl Pts',(-14.1429487704599,40.3604431105938,
42.9999999999987));
#126052=CARTESIAN_POINT('Ctrl Pts',(-14.1509424007594,40.384961681931,43.));
#126053=CARTESIAN_POINT('Origin',(16.0005712344353,40.3838853813626,66.));
#126054=CARTESIAN_POINT('',(16.0005576038968,40.0020390449739,63.0244003328805));
#126055=CARTESIAN_POINT('',(16.0005576038968,40.0020390449739,68.9755996671195));
#126056=CARTESIAN_POINT('',(16.0005576038968,40.0020390450537,46.));
#126057=CARTESIAN_POINT('Origin',(16.0005712344353,40.3838853813626,66.));
#126058=CARTESIAN_POINT('Origin',(-25.9994287388058,40.3853846300409,66.));
#126059=CARTESIAN_POINT('',(-16.000205842957,40.3850276938095,63.));
#126060=CARTESIAN_POINT('Origin',(-16.000205842957,40.3850276938095,66.));
#126061=CARTESIAN_POINT('',(-14.1509424007594,40.3849616818491,63.));
#126062=CARTESIAN_POINT('',(-25.9994287388058,40.3853846300409,63.));
#126063=CARTESIAN_POINT('',(-14.2001947782207,40.6949634400972,63.0160596520708));
#126064=CARTESIAN_POINT('Ctrl Pts',(-14.1509424007594,40.384961681931,63.));
#126065=CARTESIAN_POINT('Ctrl Pts',(-14.1842343067511,40.4870767337193,
63.0000000000056));
#126066=CARTESIAN_POINT('Ctrl Pts',(-14.2001983851187,40.5939196884095,
63.0055622696198));
#126067=CARTESIAN_POINT('Ctrl Pts',(-14.2001947782208,40.6949634400972,
63.0160596520708));
#126068=CARTESIAN_POINT('',(-14.200125669996,42.6309634388637,64.0111601371654));
#126069=CARTESIAN_POINT('Origin',(-14.2002058441038,40.3849634402947,66.));
#126070=CARTESIAN_POINT('',(-13.700107822116,43.1309455903466,64.7919089438291));
#126071=CARTESIAN_POINT('Ctrl Pts',(-13.700107822116,43.1309455903466,64.7919089438292));
#126072=CARTESIAN_POINT('Ctrl Pts',(-13.7287138176145,43.1309466114776,
64.7919089438292));
#126073=CARTESIAN_POINT('Ctrl Pts',(-13.7588198896061,43.1282901354821,
64.7858171356271));
#126074=CARTESIAN_POINT('Ctrl Pts',(-13.8150242028358,43.1184187630571,
64.7637668516514));
#126075=CARTESIAN_POINT('Ctrl Pts',(-13.8411536038327,43.1112169321056,
64.7478820248202));
#126076=CARTESIAN_POINT('Ctrl Pts',(-13.942146077159,43.0763467034421,64.6731422398801));
#126077=CARTESIAN_POINT('Ctrl Pts',(-14.0082080214715,43.0299667749565,
64.5814744645503));
#126078=CARTESIAN_POINT('Ctrl Pts',(-14.1423359864052,42.8958483854512,
64.3486366205185));
#126079=CARTESIAN_POINT('Ctrl Pts',(-14.2001209716938,42.7625818225232,
64.1597969859191));
#126080=CARTESIAN_POINT('Ctrl Pts',(-14.2001256699959,42.6309634388638,
64.0111601371654));
#126081=CARTESIAN_POINT('',(-12.8001078226894,43.1309134635892,64.7919089438291));
#126082=CARTESIAN_POINT('',(-25.9993307164994,43.1313846282914,64.7919089438291));
#126083=CARTESIAN_POINT('',(-12.8001078226894,43.1309134635892,67.2080910561709));
#126084=CARTESIAN_POINT('Ctrl Pts',(-12.8001078226893,43.1309134635892,
67.2080910561709));
#126085=CARTESIAN_POINT('Ctrl Pts',(-12.7874290218161,43.1309130110017,
67.2080910561709));
#126086=CARTESIAN_POINT('Ctrl Pts',(-12.7747450872089,43.1317310514822,
67.2062354373186));
#126087=CARTESIAN_POINT('Ctrl Pts',(-12.7501661862404,43.1348375455173,
67.199133868969));
#126088=CARTESIAN_POINT('Ctrl Pts',(-12.7382804382214,43.1371385398321,
67.193861533145));
#126089=CARTESIAN_POINT('Ctrl Pts',(-12.7046747516163,43.1455281504129,
67.1743800110828));
#126090=CARTESIAN_POINT('Ctrl Pts',(-12.6851453672407,43.1532658613644,
67.1561143770981));
#126091=CARTESIAN_POINT('Ctrl Pts',(-12.6471649980075,43.1716314784724,
67.111298056684));
#126092=CARTESIAN_POINT('Ctrl Pts',(-12.6264424973877,43.1855881094717,
67.0757741121274));
#126093=CARTESIAN_POINT('Ctrl Pts',(-12.5778499600881,43.224674918756,66.9705448594992));
#126094=CARTESIAN_POINT('Ctrl Pts',(-12.5550921166024,43.2558293923731,
66.8746617707269));
#126095=CARTESIAN_POINT('Ctrl Pts',(-12.5029059493652,43.3441575831397,
66.5522053662921));
#126096=CARTESIAN_POINT('Ctrl Pts',(-12.5036463989442,43.3849028811463,
66.2522550206409));
#126097=CARTESIAN_POINT('Ctrl Pts',(-12.5036463989442,43.3849028811463,
65.7477449793591));
#126098=CARTESIAN_POINT('Ctrl Pts',(-12.5029059493652,43.3441575831397,
65.4477946337079));
#126099=CARTESIAN_POINT('Ctrl Pts',(-12.5550921166024,43.2558293923731,
65.1253382292731));
#126100=CARTESIAN_POINT('Ctrl Pts',(-12.5778499600881,43.224674918756,65.0294551405009));
#126101=CARTESIAN_POINT('Ctrl Pts',(-12.6264424973877,43.1855881094717,
64.9242258878726));
#126102=CARTESIAN_POINT('Ctrl Pts',(-12.6471649980075,43.1716314784724,
64.888701943316));
#126103=CARTESIAN_POINT('Ctrl Pts',(-12.6851453672407,43.1532658613644,
64.8438856229019));
#126104=CARTESIAN_POINT('Ctrl Pts',(-12.7046747516163,43.1455281504129,
64.8256199889173));
#126105=CARTESIAN_POINT('Ctrl Pts',(-12.7382804382214,43.1371385398321,
64.806138466855));
#126106=CARTESIAN_POINT('Ctrl Pts',(-12.7501661862404,43.1348375455173,
64.800866131031));
#126107=CARTESIAN_POINT('Ctrl Pts',(-12.7747450872089,43.1317310514822,
64.7937645626814));
#126108=CARTESIAN_POINT('Ctrl Pts',(-12.7874290218161,43.1309130110017,
64.7919089438292));
#126109=CARTESIAN_POINT('Ctrl Pts',(-12.8001078226893,43.1309134635892,
64.7919089438292));
#126110=CARTESIAN_POINT('',(-13.700107822116,43.1309455903466,67.2080910561709));
#126111=CARTESIAN_POINT('',(-25.9993307164994,43.1313846282914,67.2080910561709));
#126112=CARTESIAN_POINT('',(-14.200125669996,42.6309634388637,67.9888398628346));
#126113=CARTESIAN_POINT('Ctrl Pts',(-14.2001256699959,42.6309634388638,
67.9888398628346));
#126114=CARTESIAN_POINT('Ctrl Pts',(-14.2001209716939,42.7625818225232,
67.8402030140809));
#126115=CARTESIAN_POINT('Ctrl Pts',(-14.1423359864052,42.8958483854512,
67.6513633794815));
#126116=CARTESIAN_POINT('Ctrl Pts',(-14.0082080214715,43.0299667749565,
67.4185255354497));
#126117=CARTESIAN_POINT('Ctrl Pts',(-13.942146077159,43.0763467034421,67.3268577601199));
#126118=CARTESIAN_POINT('Ctrl Pts',(-13.8411536038327,43.1112169321056,
67.2521179751798));
#126119=CARTESIAN_POINT('Ctrl Pts',(-13.8150242028358,43.1184187630571,
67.2362331483486));
#126120=CARTESIAN_POINT('Ctrl Pts',(-13.7588198896061,43.1282901354821,
67.2141828643729));
#126121=CARTESIAN_POINT('Ctrl Pts',(-13.7287138176144,43.1309466114776,
67.2080910561708));
#126122=CARTESIAN_POINT('Ctrl Pts',(-13.7001078221159,43.1309455903466,
67.2080910561708));
#126123=CARTESIAN_POINT('',(-14.2001947782207,40.6949634400972,68.9839403479292));
#126124=CARTESIAN_POINT('Origin',(-14.2002058441038,40.3849634402947,66.));
#126125=CARTESIAN_POINT('',(-13.9073268007583,39.9878462041285,68.9736015544009));
#126126=CARTESIAN_POINT('Ctrl Pts',(-13.9073268007584,39.9878462041285,
68.973601554401));
#126127=CARTESIAN_POINT('Ctrl Pts',(-13.9960100566734,40.076535791615,68.9854450979406));
#126128=CARTESIAN_POINT('Ctrl Pts',(-14.0730534099154,40.1890412751135,
68.9961344807684));
#126129=CARTESIAN_POINT('Ctrl Pts',(-14.1751560019799,40.435594122051,69.0021062582817));
#126130=CARTESIAN_POINT('Ctrl Pts',(-14.2001992511613,40.5696583440676,
68.9969582287394));
#126131=CARTESIAN_POINT('Ctrl Pts',(-14.2001947782208,40.6949634400972,
68.9839403479292));
#126132=CARTESIAN_POINT('',(-13.0856980517762,39.1661587946801,68.7412793024013));
#126133=CARTESIAN_POINT('Origin',(-14.3044194064105,40.3849671603434,66.));
#126134=CARTESIAN_POINT('',(-11.6715054007694,38.5803218750975,68.3965797735301));
#126135=CARTESIAN_POINT('Ctrl Pts',(-11.6715054007694,38.5803218750975,
68.3965797735301));
#126136=CARTESIAN_POINT('Ctrl Pts',(-11.9310804859103,38.5803311409929,
68.3965797735301));
#126137=CARTESIAN_POINT('Ctrl Pts',(-12.2008654839661,38.6335041042047,
68.4388004161354));
#126138=CARTESIAN_POINT('Ctrl Pts',(-12.6901619533851,38.8388876989633,
68.5738923324279));
#126139=CARTESIAN_POINT('Ctrl Pts',(-12.9106059326522,38.9910541747943,
68.6634310729608));
#126140=CARTESIAN_POINT('Ctrl Pts',(-13.0856980517762,39.1661587946801,
68.7412793024013));
#126141=CARTESIAN_POINT('',(-9.57050540210797,38.5802468769672,68.39657977353));
#126142=CARTESIAN_POINT('',(-25.9994931547856,38.5808333326384,68.3965797735301));
#126143=CARTESIAN_POINT('',(-6.03491922226453,40.0445867642791,68.980661345019));
#126144=CARTESIAN_POINT('Ctrl Pts',(-6.03491922226454,40.0445867642791,
68.980661345019));
#126145=CARTESIAN_POINT('Ctrl Pts',(-6.46491979272285,39.6146168916673,
68.9316012220604));
#126146=CARTESIAN_POINT('Ctrl Pts',(-6.98352950944328,39.2568425175939,
68.7941482303742));
#126147=CARTESIAN_POINT('Ctrl Pts',(-8.18737580567769,38.7250267702563,
68.519101496493));
#126148=CARTESIAN_POINT('Ctrl Pts',(-8.88897256914252,38.5802225487005,
68.39657977353));
#126149=CARTESIAN_POINT('Ctrl Pts',(-9.57050540210795,38.5802468769672,
68.39657977353));
#126150=CARTESIAN_POINT('',(-4.31517414500253,41.7642090685172,68.6639647170472));
#126151=CARTESIAN_POINT('Origin',(-5.69482187817972,40.3846598287309,66.));
#126152=CARTESIAN_POINT('',(-4.88081081954212,43.1299146855279,67.2097174218851));
#126153=CARTESIAN_POINT('Ctrl Pts',(-4.88081081954212,43.1299146855279,
67.2097174218852));
#126154=CARTESIAN_POINT('Ctrl Pts',(-4.82482221472671,43.1299126869364,
67.2097174218852));
#126155=CARTESIAN_POINT('Ctrl Pts',(-4.77320031795728,43.1241916785181,
67.2228273668612));
#126156=CARTESIAN_POINT('Ctrl Pts',(-4.67621148812539,43.104869821818,67.2652368623581));
#126157=CARTESIAN_POINT('Ctrl Pts',(-4.63083615831867,43.0912259898174,
67.2944976062002));
#126158=CARTESIAN_POINT('Ctrl Pts',(-4.5029953131025,43.0409837535405,67.3962229005734));
#126159=CARTESIAN_POINT('Ctrl Pts',(-4.42918588082232,42.9947395232464,
67.4819738279894));
#126160=CARTESIAN_POINT('Ctrl Pts',(-4.28473708613121,42.8747600616692,
67.6785381778342));
#126161=CARTESIAN_POINT('Ctrl Pts',(-4.21173521992966,42.7838888359608,
67.808410822416));
#126162=CARTESIAN_POINT('Ctrl Pts',(-4.10948896604543,42.5724250222423,
68.0592085197964));
#126163=CARTESIAN_POINT('Ctrl Pts',(-4.08083503287425,42.4515873535033,
68.1801672395615));
#126164=CARTESIAN_POINT('Ctrl Pts',(-4.08084269258332,42.2370080209205,
68.3629383226615));
#126165=CARTESIAN_POINT('Ctrl Pts',(-4.09805029004739,42.1312231898084,
68.4421976606013));
#126166=CARTESIAN_POINT('Ctrl Pts',(-4.17859647402362,41.9330114055893,
68.5720688356092));
#126167=CARTESIAN_POINT('Ctrl Pts',(-4.23902256544591,41.8403552115938,
68.6245291895113));
#126168=CARTESIAN_POINT('Ctrl Pts',(-4.31517414500254,41.7642090685172,
68.6639647170472));
#126169=CARTESIAN_POINT('',(-7.19981081806464,43.1299974654728,67.209717421885));
#126170=CARTESIAN_POINT('',(-25.9993307420611,43.1306685406019,67.2097174218847));
#126171=CARTESIAN_POINT('',(-7.19981081806464,43.1299974654728,64.790282578115));
#126172=CARTESIAN_POINT('Ctrl Pts',(-7.19981081806464,43.1299974654728,
64.790282578115));
#126173=CARTESIAN_POINT('Ctrl Pts',(-7.21250680486427,43.1299979186738,
64.790282578115));
#126174=CARTESIAN_POINT('Ctrl Pts',(-7.22520787530932,43.1308190809083,
64.7921402324464));
#126175=CARTESIAN_POINT('Ctrl Pts',(-7.24981968793656,43.1339357989149,
64.7992497365214));
#126176=CARTESIAN_POINT('Ctrl Pts',(-7.26172119707253,43.13624393064,64.8045280031557));
#126177=CARTESIAN_POINT('Ctrl Pts',(-7.29537069273696,43.1446590481209,
64.8240319462818));
#126178=CARTESIAN_POINT('Ctrl Pts',(-7.31492435500479,43.1524197100444,
64.8423192550511));
#126179=CARTESIAN_POINT('Ctrl Pts',(-7.35294574461562,43.1708382902919,
64.8871870557474));
#126180=CARTESIAN_POINT('Ctrl Pts',(-7.37368596111585,43.1848338692446,
64.9227502546591));
#126181=CARTESIAN_POINT('Ctrl Pts',(-7.42230928437433,43.2240280671579,
65.0280938938583));
#126182=CARTESIAN_POINT('Ctrl Pts',(-7.44506219926235,43.2552667477377,
65.1240810706962));
#126183=CARTESIAN_POINT('Ctrl Pts',(-7.49721225591251,43.34385822923,65.4469741746507));
#126184=CARTESIAN_POINT('Ctrl Pts',(-7.49636431121142,43.3847241392164,
65.7473663615792));
#126185=CARTESIAN_POINT('Ctrl Pts',(-7.49636431121142,43.3847241392164,
66.2526336384208));
#126186=CARTESIAN_POINT('Ctrl Pts',(-7.49721225591251,43.34385822923,66.5530258253493));
#126187=CARTESIAN_POINT('Ctrl Pts',(-7.44506219926235,43.2552667477377,
66.8759189293038));
#126188=CARTESIAN_POINT('Ctrl Pts',(-7.42230928437433,43.2240280671579,
66.9719061061417));
#126189=CARTESIAN_POINT('Ctrl Pts',(-7.37368596111585,43.1848338692446,
67.0772497453409));
#126190=CARTESIAN_POINT('Ctrl Pts',(-7.35294574461562,43.1708382902919,
67.1128129442526));
#126191=CARTESIAN_POINT('Ctrl Pts',(-7.31492435500479,43.1524197100444,
67.1576807449489));
#126192=CARTESIAN_POINT('Ctrl Pts',(-7.29537069273696,43.1446590481209,
67.1759680537182));
#126193=CARTESIAN_POINT('Ctrl Pts',(-7.26172119707253,43.13624393064,67.1954719968443));
#126194=CARTESIAN_POINT('Ctrl Pts',(-7.24981968793656,43.1339357989149,
67.2007502634786));
#126195=CARTESIAN_POINT('Ctrl Pts',(-7.22520787530932,43.1308190809083,
67.2078597675536));
#126196=CARTESIAN_POINT('Ctrl Pts',(-7.21250680486427,43.1299979186738,
67.209717421885));
#126197=CARTESIAN_POINT('Ctrl Pts',(-7.19981081806464,43.1299974654728,
67.209717421885));
#126198=CARTESIAN_POINT('',(-4.88081081954212,43.1299146855279,64.7902825781149));
#126199=CARTESIAN_POINT('',(-25.9993307420611,43.1306685406019,64.7902825781153));
#126200=CARTESIAN_POINT('',(-4.31517414500253,41.7642090685172,63.3360352829528));
#126201=CARTESIAN_POINT('Ctrl Pts',(-4.31517414500255,41.7642090685172,
63.3360352829528));
#126202=CARTESIAN_POINT('Ctrl Pts',(-4.23902256544591,41.8403552115938,
63.3754708104887));
#126203=CARTESIAN_POINT('Ctrl Pts',(-4.17859647402362,41.9330114055893,
63.4279311643908));
#126204=CARTESIAN_POINT('Ctrl Pts',(-4.09805029004739,42.1312231898084,
63.5578023393987));
#126205=CARTESIAN_POINT('Ctrl Pts',(-4.08084269258332,42.2370080209205,
63.6370616773385));
#126206=CARTESIAN_POINT('Ctrl Pts',(-4.08083503287425,42.4515873535033,
63.8198327604385));
#126207=CARTESIAN_POINT('Ctrl Pts',(-4.10948896604543,42.5724250222423,
63.9407914802036));
#126208=CARTESIAN_POINT('Ctrl Pts',(-4.21173521992966,42.7838888359608,
64.191589177584));
#126209=CARTESIAN_POINT('Ctrl Pts',(-4.28473708613121,42.8747600616692,
64.3214618221658));
#126210=CARTESIAN_POINT('Ctrl Pts',(-4.42918588082232,42.9947395232464,
64.5180261720106));
#126211=CARTESIAN_POINT('Ctrl Pts',(-4.50299531310249,43.0409837535405,
64.6037770994266));
#126212=CARTESIAN_POINT('Ctrl Pts',(-4.63083615831866,43.0912259898174,
64.7055023937998));
#126213=CARTESIAN_POINT('Ctrl Pts',(-4.67621148812537,43.104869821818,64.7347631376419));
#126214=CARTESIAN_POINT('Ctrl Pts',(-4.77320031795728,43.1241916785181,
64.7771726331388));
#126215=CARTESIAN_POINT('Ctrl Pts',(-4.82482221472671,43.1299126869364,
64.7902825781148));
#126216=CARTESIAN_POINT('Ctrl Pts',(-4.88081081954212,43.1299146855279,
64.7902825781148));
#126217=CARTESIAN_POINT('',(-5.69482187817968,40.384659828731,63.));
#126218=CARTESIAN_POINT('Origin',(-5.69482187817972,40.3846598287309,66.));
#126219=CARTESIAN_POINT('',(5.69537693071232,40.384253239671,63.));
#126220=CARTESIAN_POINT('',(-25.9994287388058,40.3853846300409,63.));
#126221=CARTESIAN_POINT('',(4.3155751451931,41.7640550251902,63.3361150636597));
#126222=CARTESIAN_POINT('Origin',(5.69537693071237,40.3842532396709,66.));
#126223=CARTESIAN_POINT('',(4.88126057014233,43.1297404501394,64.7906780580687));
#126224=CARTESIAN_POINT('Ctrl Pts',(4.88126057014233,43.1297404501394,64.7906780580686));
#126225=CARTESIAN_POINT('Ctrl Pts',(4.82527855129633,43.1297404501394,64.7906735213083));
#126226=CARTESIAN_POINT('Ctrl Pts',(4.77366641546815,43.1240229215084,64.7775580917314));
#126227=CARTESIAN_POINT('Ctrl Pts',(4.6766881693441,43.1047100794269,64.7351374178226));
#126228=CARTESIAN_POINT('Ctrl Pts',(4.63131473335929,43.0910704365374,64.7058682945448));
#126229=CARTESIAN_POINT('Ctrl Pts',(4.50347730469684,43.040841140764,64.6041166977585));
#126230=CARTESIAN_POINT('Ctrl Pts',(4.42966809762419,42.9946063244288,64.5183478507339));
#126231=CARTESIAN_POINT('Ctrl Pts',(4.28521059479939,42.8746430433406,64.3217402796909));
#126232=CARTESIAN_POINT('Ctrl Pts',(4.21219885970608,42.7837779689826,64.1918390912013));
#126233=CARTESIAN_POINT('Ctrl Pts',(4.10993073305515,42.5723177386493,63.9409875062198));
#126234=CARTESIAN_POINT('Ctrl Pts',(4.08126491520575,42.4514774729932,63.8200033709792));
#126235=CARTESIAN_POINT('Ctrl Pts',(4.08125725528774,42.2368922872938,63.6371990515189));
#126236=CARTESIAN_POINT('Ctrl Pts',(4.09845674449903,42.1311064778841,63.5579277928478));
#126237=CARTESIAN_POINT('Ctrl Pts',(4.17899207419104,41.9328803074183,63.4280312090116));
#126238=CARTESIAN_POINT('Ctrl Pts',(4.23941854432905,41.8402116260542,63.375558776258));
#126239=CARTESIAN_POINT('Ctrl Pts',(4.31557514519307,41.7640550251902,63.3361150636597));
#126240=CARTESIAN_POINT('',(7.20026057014233,43.1297404501395,64.7908660063353));
#126241=CARTESIAN_POINT('',(6.04076057014233,43.1297404501395,64.790772032202));
#126242=CARTESIAN_POINT('',(7.20026057014233,43.1297404501395,67.2091339936647));
#126243=CARTESIAN_POINT('Ctrl Pts',(7.20026057014233,43.1297404501395,67.2091339936646));
#126244=CARTESIAN_POINT('Ctrl Pts',(7.21294682501949,43.1297404501395,67.2091329653848));
#126245=CARTESIAN_POINT('Ctrl Pts',(7.22563810372133,43.1305598955788,67.2072760701667));
#126246=CARTESIAN_POINT('Ctrl Pts',(7.25023479260246,43.1336713801016,67.2001704115751));
#126247=CARTESIAN_POINT('Ctrl Pts',(7.26213075345329,43.1359764055222,67.1948942718855));
#126248=CARTESIAN_POINT('Ctrl Pts',(7.29576491915057,43.144380828481,67.1753983698309));
#126249=CARTESIAN_POINT('Ctrl Pts',(7.31531022822448,43.152132358212,67.1571188348341));
#126250=CARTESIAN_POINT('Ctrl Pts',(7.35331775020092,43.1705301900497,67.1122694969576));
#126251=CARTESIAN_POINT('Ctrl Pts',(7.3740522567382,43.1845108420159,67.0767203752738));
#126252=CARTESIAN_POINT('Ctrl Pts',(7.4226663467744,43.2236642757062,66.9714177547315));
#126253=CARTESIAN_POINT('Ctrl Pts',(7.44542247694709,43.2548716957552,66.8754679026737));
#126254=CARTESIAN_POINT('Ctrl Pts',(7.49758960390303,43.3433662832606,66.5527314566462));
#126255=CARTESIAN_POINT('Ctrl Pts',(7.49678217092917,43.3841889379055,66.2524977920887));
#126256=CARTESIAN_POINT('Ctrl Pts',(7.49678217092917,43.3841889379055,65.7475022079113));
#126257=CARTESIAN_POINT('Ctrl Pts',(7.49758960390303,43.3433662832606,65.4472685433538));
#126258=CARTESIAN_POINT('Ctrl Pts',(7.44542247694709,43.2548716957552,65.1245320973263));
#126259=CARTESIAN_POINT('Ctrl Pts',(7.4226663467744,43.2236642757062,65.0285822452685));
#126260=CARTESIAN_POINT('Ctrl Pts',(7.3740522567382,43.1845108420159,64.9232796247263));
#126261=CARTESIAN_POINT('Ctrl Pts',(7.35331775020091,43.1705301900497,64.8877305030424));
#126262=CARTESIAN_POINT('Ctrl Pts',(7.31531022822448,43.152132358212,64.8428811651659));
#126263=CARTESIAN_POINT('Ctrl Pts',(7.29576491915057,43.144380828481,64.8246016301691));
#126264=CARTESIAN_POINT('Ctrl Pts',(7.26213075345329,43.1359764055222,64.8051057281145));
#126265=CARTESIAN_POINT('Ctrl Pts',(7.25023479260246,43.1336713801016,64.7998295884249));
#126266=CARTESIAN_POINT('Ctrl Pts',(7.22563810372133,43.1305598955788,64.7927239298334));
#126267=CARTESIAN_POINT('Ctrl Pts',(7.21294682501949,43.1297404501395,64.7908670346152));
#126268=CARTESIAN_POINT('Ctrl Pts',(7.20026057014233,43.1297404501395,64.7908660063354));
#126269=CARTESIAN_POINT('',(4.88126057014233,43.1297404501394,67.2093219419313));
#126270=CARTESIAN_POINT('',(6.04076057014233,43.1297404501395,67.209227967798));
#126271=CARTESIAN_POINT('',(4.3155751451931,41.7640550251902,68.6638849363403));
#126272=CARTESIAN_POINT('Ctrl Pts',(4.31557514519307,41.7640550251902,68.6638849363403));
#126273=CARTESIAN_POINT('Ctrl Pts',(4.23941854432905,41.8402116260542,68.624441223742));
#126274=CARTESIAN_POINT('Ctrl Pts',(4.17899207419104,41.9328803074183,68.5719687909884));
#126275=CARTESIAN_POINT('Ctrl Pts',(4.09845674449903,42.1311064778841,68.4420722071522));
#126276=CARTESIAN_POINT('Ctrl Pts',(4.08125725528774,42.2368922872938,68.3628009484811));
#126277=CARTESIAN_POINT('Ctrl Pts',(4.08126491520575,42.4514774729932,68.1799966290208));
#126278=CARTESIAN_POINT('Ctrl Pts',(4.10993073305515,42.5723177386493,68.0590124937802));
#126279=CARTESIAN_POINT('Ctrl Pts',(4.21219885970608,42.7837779689826,67.8081609087987));
#126280=CARTESIAN_POINT('Ctrl Pts',(4.28521059479939,42.8746430433406,67.6782597203091));
#126281=CARTESIAN_POINT('Ctrl Pts',(4.42966809762419,42.9946063244288,67.4816521492661));
#126282=CARTESIAN_POINT('Ctrl Pts',(4.50347730469684,43.040841140764,67.3958833022415));
#126283=CARTESIAN_POINT('Ctrl Pts',(4.63131473335929,43.0910704365374,67.2941317054552));
#126284=CARTESIAN_POINT('Ctrl Pts',(4.6766881693441,43.1047100794269,67.2648625821774));
#126285=CARTESIAN_POINT('Ctrl Pts',(4.77366641546815,43.1240229215084,67.2224419082686));
#126286=CARTESIAN_POINT('Ctrl Pts',(4.82527855129632,43.1297404501394,67.2093264786917));
#126287=CARTESIAN_POINT('Ctrl Pts',(4.88126057014233,43.1297404501394,67.2093219419314));
#126288=CARTESIAN_POINT('',(6.03525883703878,40.0443713333445,68.9806859172054));
#126289=CARTESIAN_POINT('Origin',(5.69537693071237,40.3842532396709,66.));
#126290=CARTESIAN_POINT('',(9.57079274297153,38.5799052392773,68.3968369781133));
#126291=CARTESIAN_POINT('Ctrl Pts',(9.57079274297153,38.5799052392773,68.3968369781133));
#126292=CARTESIAN_POINT('Ctrl Pts',(9.5707332488234,38.5799052392773,68.3968369765146));
#126293=CARTESIAN_POINT('Ctrl Pts',(9.5706737548282,38.5799052403392,68.3968369757153));
#126294=CARTESIAN_POINT('Ctrl Pts',(8.88909486927775,38.5799295702497,68.3968369757153));
#126295=CARTESIAN_POINT('Ctrl Pts',(8.1875100639932,38.724779883745,68.5193208964011));
#126296=CARTESIAN_POINT('Ctrl Pts',(6.98374971135328,39.2566553618154,68.7942694455703));
#126297=CARTESIAN_POINT('Ctrl Pts',(6.46520448621751,39.6144256841658,68.9316635383853));
#126298=CARTESIAN_POINT('Ctrl Pts',(6.03525883703881,40.0443713333445,68.9806859172054));
#126299=CARTESIAN_POINT('',(11.6717927429715,38.5799052392773,68.3968934308243));
#126300=CARTESIAN_POINT('',(10.6212927429715,38.5799052392773,68.3968652044688));
#126301=CARTESIAN_POINT('',(13.0860063053446,39.1656916769042,68.7414869339534));
#126302=CARTESIAN_POINT('Ctrl Pts',(13.0860063053446,39.1656916769042,68.7414869339534));
#126303=CARTESIAN_POINT('Ctrl Pts',(12.9115776150688,38.9912629866284,68.663969269128));
#126304=CARTESIAN_POINT('Ctrl Pts',(12.6925492447761,38.8399015743528,68.5750351340623));
#126305=CARTESIAN_POINT('Ctrl Pts',(12.2039210685268,38.6336428861301,68.4395838913209));
#126306=CARTESIAN_POINT('Ctrl Pts',(11.9328135534399,38.5799052392773,68.3969004440812));
#126307=CARTESIAN_POINT('Ctrl Pts',(11.6717927429715,38.5799052392773,68.3968934308244));
#126308=CARTESIAN_POINT('',(13.9076643850834,39.987349756643,68.973667809827));
#126309=CARTESIAN_POINT('Origin',(14.3042605619825,40.383945933542,66.));
#126310=CARTESIAN_POINT('',(14.2005576038968,40.6944565378947,68.9838876432241));
#126311=CARTESIAN_POINT('Ctrl Pts',(14.2005576038968,40.6944565378295,68.9838876425972));
#126312=CARTESIAN_POINT('Ctrl Pts',(14.2005576038968,40.6944446389709,68.9838888808066));
#126313=CARTESIAN_POINT('Ctrl Pts',(14.2005576036844,40.6944327401719,68.9838901189378));
#126314=CARTESIAN_POINT('Ctrl Pts',(14.2005531444961,40.5695128967916,68.996887916041));
#126315=CARTESIAN_POINT('Ctrl Pts',(14.1756575752172,40.4358460629751,69.0020722846323));
#126316=CARTESIAN_POINT('Ctrl Pts',(14.0741268986634,40.1899012740497,68.9962434199587));
#126317=CARTESIAN_POINT('Ctrl Pts',(13.9975074091711,40.0776069665203,68.9856559212044));
#126318=CARTESIAN_POINT('Ctrl Pts',(13.9087580506029,39.988444692808,68.9738136974118));
#126319=CARTESIAN_POINT('Ctrl Pts',(13.9082116449317,39.9878970164913,68.9737408027343));
#126320=CARTESIAN_POINT('Ctrl Pts',(13.9076643850834,39.987349756643,68.973667809827));
#126321=CARTESIAN_POINT('',(14.2005576038968,42.6304565378295,67.9882672716729));
#126322=CARTESIAN_POINT('Origin',(14.2005576038968,40.383949635364,66.));
#126323=CARTESIAN_POINT('',(13.7005576038968,43.1304565378295,67.2069788251679));
#126324=CARTESIAN_POINT('Ctrl Pts',(13.7005576038968,43.1304565378295,67.206978825168));
#126325=CARTESIAN_POINT('Ctrl Pts',(13.7005635533611,43.1304565378295,67.2069788246847));
#126326=CARTESIAN_POINT('Ctrl Pts',(13.7005695027606,43.1304565377233,67.2069788244431));
#126327=CARTESIAN_POINT('Ctrl Pts',(13.7349434333177,43.1304553106978,67.2069788244431));
#126328=CARTESIAN_POINT('Ctrl Pts',(13.7667215268191,43.1269938687308,67.2149030662356));
#126329=CARTESIAN_POINT('Ctrl Pts',(13.8263020113281,43.1153320791706,67.240899990775));
#126330=CARTESIAN_POINT('Ctrl Pts',(13.8540993385831,43.1071092325231,67.2589741809338));
#126331=CARTESIAN_POINT('Ctrl Pts',(13.9319395673727,43.0771707831725,67.3224216534088));
#126332=CARTESIAN_POINT('Ctrl Pts',(13.9761986813102,43.0500508066361,67.3767434803275));
#126333=CARTESIAN_POINT('Ctrl Pts',(14.070024541769,42.9755247782782,67.5143570677025));
#126334=CARTESIAN_POINT('Ctrl Pts',(14.1174300227276,42.916521123884,67.6124763023577));
#126335=CARTESIAN_POINT('Ctrl Pts',(14.1829744042219,42.7817463851036,67.8068079086529));
#126336=CARTESIAN_POINT('Ctrl Pts',(14.2005576038968,42.7058286960662,67.9031056458045));
#126337=CARTESIAN_POINT('Ctrl Pts',(14.2005576038968,42.6304565378295,67.9882672716729));
#126338=CARTESIAN_POINT('',(12.8005576038968,43.1304565378295,67.2070519271956));
#126339=CARTESIAN_POINT('',(13.2505576038968,43.1304565378295,67.2070153761818));
#126340=CARTESIAN_POINT('',(12.8005576038968,43.1304565378295,64.7929480728044));
#126341=CARTESIAN_POINT('Ctrl Pts',(12.8005576038968,43.1304565378295,64.7929480728044));
#126342=CARTESIAN_POINT('Ctrl Pts',(12.8005540342567,43.1304565378295,64.7929480725144));
#126343=CARTESIAN_POINT('Ctrl Pts',(12.800550464617,43.1304565378932,64.7929480723695));
#126344=CARTESIAN_POINT('Ctrl Pts',(12.8005468949777,43.1304565380206,64.7929480723695));
#126345=CARTESIAN_POINT('Ctrl Pts',(12.7878790745653,43.1304569902162,64.7929480723695));
#126346=CARTESIAN_POINT('Ctrl Pts',(12.775206184161,43.1312745218071,64.7948023896052));
#126347=CARTESIAN_POINT('Ctrl Pts',(12.7506486750991,43.1343773655443,64.801898883713));
#126348=CARTESIAN_POINT('Ctrl Pts',(12.738773266856,43.1366751949132,64.8071674273607));
#126349=CARTESIAN_POINT('Ctrl Pts',(12.7051965550664,43.1450524580709,64.826634614644));
#126350=CARTESIAN_POINT('Ctrl Pts',(12.6856835914487,43.1527778071505,64.8448863925531));
#126351=CARTESIAN_POINT('Ctrl Pts',(12.6477316006356,43.1711140657731,64.8896697992273));
#126352=CARTESIAN_POINT('Ctrl Pts',(12.6270220730305,43.1850482619964,64.9251686425469));
#126353=CARTESIAN_POINT('Ctrl Pts',(12.5784538537086,43.2240722091775,65.0303247407441));
#126354=CARTESIAN_POINT('Ctrl Pts',(12.5556965844494,43.2551755942419,65.126141257432));
#126355=CARTESIAN_POINT('Ctrl Pts',(12.5034979555493,43.3433419209884,65.4483186441275));
#126356=CARTESIAN_POINT('Ctrl Pts',(12.5041748497398,43.3840101920279,65.7479867774995));
#126357=CARTESIAN_POINT('Ctrl Pts',(12.5041748497398,43.3840101920279,66.2520132225005));
#126358=CARTESIAN_POINT('Ctrl Pts',(12.5034979555493,43.3433419209884,66.5516813558725));
#126359=CARTESIAN_POINT('Ctrl Pts',(12.5556965844494,43.2551755942419,66.873858742568));
#126360=CARTESIAN_POINT('Ctrl Pts',(12.5784538537086,43.2240722091775,66.9696752592559));
#126361=CARTESIAN_POINT('Ctrl Pts',(12.6270220730305,43.1850482619964,67.0748313574531));
#126362=CARTESIAN_POINT('Ctrl Pts',(12.6477316006356,43.1711140657731,67.1103302007727));
#126363=CARTESIAN_POINT('Ctrl Pts',(12.6856835914487,43.1527778071505,67.1551136074469));
#126364=CARTESIAN_POINT('Ctrl Pts',(12.7051965550664,43.1450524580709,67.173365385356));
#126365=CARTESIAN_POINT('Ctrl Pts',(12.738773266856,43.1366751949132,67.1928325726393));
#126366=CARTESIAN_POINT('Ctrl Pts',(12.7506486750991,43.1343773655443,67.198101116287));
#126367=CARTESIAN_POINT('Ctrl Pts',(12.775206184161,43.1312745218071,67.2051976103948));
#126368=CARTESIAN_POINT('Ctrl Pts',(12.7878790745653,43.1304569902162,67.2070519276305));
#126369=CARTESIAN_POINT('Ctrl Pts',(12.800550464617,43.1304565378932,67.2070519276305));
#126370=CARTESIAN_POINT('Ctrl Pts',(12.8005540342567,43.1304565378295,67.2070519274856));
#126371=CARTESIAN_POINT('Ctrl Pts',(12.8005576038968,43.1304565378295,67.2070519271956));
#126372=CARTESIAN_POINT('',(13.7005576038968,43.1304565378295,64.7930211748321));
#126373=CARTESIAN_POINT('',(13.2505576038968,43.1304565378295,64.7929846238182));
#126374=CARTESIAN_POINT('',(14.2005576038968,42.6304565378295,64.0117327283271));
#126375=CARTESIAN_POINT('Ctrl Pts',(14.2005576038968,42.6304565378295,64.0117327283271));
#126376=CARTESIAN_POINT('Ctrl Pts',(14.2005576038968,42.7058286960662,64.0968943541956));
#126377=CARTESIAN_POINT('Ctrl Pts',(14.1829744042219,42.7817463851036,64.1931920913471));
#126378=CARTESIAN_POINT('Ctrl Pts',(14.1174300227276,42.916521123884,64.3875236976423));
#126379=CARTESIAN_POINT('Ctrl Pts',(14.070024541769,42.9755247782782,64.4856429322975));
#126380=CARTESIAN_POINT('Ctrl Pts',(13.9761986813102,43.0500508066361,64.6232565196725));
#126381=CARTESIAN_POINT('Ctrl Pts',(13.9319395673727,43.0771707831725,64.6775783465912));
#126382=CARTESIAN_POINT('Ctrl Pts',(13.8540993385831,43.1071092325231,64.7410258190662));
#126383=CARTESIAN_POINT('Ctrl Pts',(13.8263020113281,43.1153320791706,64.759100009225));
#126384=CARTESIAN_POINT('Ctrl Pts',(13.7667215268191,43.1269938687308,64.7850969337644));
#126385=CARTESIAN_POINT('Ctrl Pts',(13.7349434333177,43.1304553106978,64.7930211755569));
#126386=CARTESIAN_POINT('Ctrl Pts',(13.7005695027606,43.1304565377233,64.7930211755569));
#126387=CARTESIAN_POINT('Ctrl Pts',(13.7005635533611,43.1304565378295,64.7930211753153));
#126388=CARTESIAN_POINT('Ctrl Pts',(13.7005576038968,43.1304565378295,64.793021174832));
#126389=CARTESIAN_POINT('',(14.2005576038968,40.6944565378947,63.0161123567759));
#126390=CARTESIAN_POINT('Origin',(14.2005576038968,40.383949635364,66.));
#126391=CARTESIAN_POINT('',(14.1511293052103,40.3839513998532,63.));
#126392=CARTESIAN_POINT('Ctrl Pts',(14.1511293052103,40.3839513999301,63.));
#126393=CARTESIAN_POINT('Ctrl Pts',(14.184533612433,40.4862144071147,63.0000000000053));
#126394=CARTESIAN_POINT('Ctrl Pts',(14.2005539915515,40.5932423327881,63.0055811103851));
#126395=CARTESIAN_POINT('Ctrl Pts',(14.2005576036844,40.6944327401719,63.0161098810622));
#126396=CARTESIAN_POINT('Ctrl Pts',(14.2005576038968,40.6944446389709,63.0161111191934));
#126397=CARTESIAN_POINT('Ctrl Pts',(14.2005576038968,40.6944565378295,63.0161123574028));
#126398=CARTESIAN_POINT('',(16.0005576038968,40.3838853818492,62.9999999980887));
#126399=CARTESIAN_POINT('',(-25.9994287388058,40.3853846300409,63.));
#126400=CARTESIAN_POINT('Origin',(16.0005576038968,40.3838853818492,66.));
#126401=CARTESIAN_POINT('Origin',(16.0005576038968,40.3838853818492,66.));
#126402=CARTESIAN_POINT('',(13.9076643850834,39.987349756643,63.026332190173));
#126403=CARTESIAN_POINT('Ctrl Pts',(13.9076643850834,39.987349756643,63.026332190173));
#126404=CARTESIAN_POINT('Ctrl Pts',(13.9082116449317,39.9878970164913,63.0262591972657));
#126405=CARTESIAN_POINT('Ctrl Pts',(13.9087580506029,39.988444692808,63.0261863025882));
#126406=CARTESIAN_POINT('Ctrl Pts',(13.9975074091711,40.0776069665203,63.0143440787957));
#126407=CARTESIAN_POINT('Ctrl Pts',(14.0741268986634,40.1899012740497,63.0037565800413));
#126408=CARTESIAN_POINT('Ctrl Pts',(14.1345364020809,40.3362353976012,63.0002884772731));
#126409=CARTESIAN_POINT('Ctrl Pts',(14.1432949797111,40.3599676160584,62.9999999999988));
#126410=CARTESIAN_POINT('Ctrl Pts',(14.1511293052103,40.3839513999301,63.));
#126411=CARTESIAN_POINT('',(13.0860063053446,39.1656916769042,63.2585130660466));
#126412=CARTESIAN_POINT('Origin',(14.3042605619825,40.383945933542,66.));
#126413=CARTESIAN_POINT('',(11.6717927429715,38.5799052392773,63.6031065691757));
#126414=CARTESIAN_POINT('Ctrl Pts',(11.6717927429715,38.5799052392773,63.6031065691757));
#126415=CARTESIAN_POINT('Ctrl Pts',(11.9328135534399,38.5799052392773,63.6030995559188));
#126416=CARTESIAN_POINT('Ctrl Pts',(12.2039210685268,38.6336428861301,63.5604161086791));
#126417=CARTESIAN_POINT('Ctrl Pts',(12.6925492447761,38.8399015743528,63.4249648659377));
#126418=CARTESIAN_POINT('Ctrl Pts',(12.9115776150688,38.9912629866284,63.3360307308721));
#126419=CARTESIAN_POINT('Ctrl Pts',(13.0860063053446,39.1656916769042,63.2585130660466));
#126420=CARTESIAN_POINT('',(9.57079274297153,38.5799052392773,63.6031630218867));
#126421=CARTESIAN_POINT('',(10.6212927429715,38.5799052392773,63.6031347955312));
#126422=CARTESIAN_POINT('',(6.03525883703878,40.0443713333445,63.0193140827946));
#126423=CARTESIAN_POINT('Ctrl Pts',(6.03525883703881,40.0443713333445,63.0193140827946));
#126424=CARTESIAN_POINT('Ctrl Pts',(6.4652044862175,39.6144256841659,63.0683364616148));
#126425=CARTESIAN_POINT('Ctrl Pts',(6.98374971135328,39.2566553618154,63.2057305544297));
#126426=CARTESIAN_POINT('Ctrl Pts',(8.1875100639932,38.724779883745,63.480679103599));
#126427=CARTESIAN_POINT('Ctrl Pts',(8.88909486927775,38.5799295702497,63.6031630242847));
#126428=CARTESIAN_POINT('Ctrl Pts',(9.570614260986,38.5799052424629,63.6031630242847));
#126429=CARTESIAN_POINT('Ctrl Pts',(9.5706737548282,38.5799052403392,63.6031630242847));
#126430=CARTESIAN_POINT('Ctrl Pts',(9.5707332488234,38.5799052392773,63.6031630234854));
#126431=CARTESIAN_POINT('Ctrl Pts',(9.57079274297153,38.5799052392773,63.6031630218867));
#126432=CARTESIAN_POINT('Origin',(5.69537693071237,40.3842532396709,66.));
#126433=CARTESIAN_POINT('',(-6.03491922226453,40.0445867642791,63.019338654981));
#126434=CARTESIAN_POINT('Origin',(-5.69482187817972,40.3846598287309,66.));
#126435=CARTESIAN_POINT('',(-9.57050540210797,38.5802468769672,63.6034202264699));
#126436=CARTESIAN_POINT('Ctrl Pts',(-9.57050540210795,38.5802468769672,
63.60342022647));
#126437=CARTESIAN_POINT('Ctrl Pts',(-8.88897256914252,38.5802225487005,
63.60342022647));
#126438=CARTESIAN_POINT('Ctrl Pts',(-8.18737580567769,38.7250267702563,
63.480898503507));
#126439=CARTESIAN_POINT('Ctrl Pts',(-6.98352950944327,39.2568425175939,
63.2058517696258));
#126440=CARTESIAN_POINT('Ctrl Pts',(-6.46491979272285,39.6146168916673,
63.0683987779396));
#126441=CARTESIAN_POINT('Ctrl Pts',(-6.03491922226453,40.0445867642791,
63.019338654981));
#126442=CARTESIAN_POINT('',(-11.6715054007694,38.5803218750975,63.6034202264699));
#126443=CARTESIAN_POINT('',(-25.9994931547856,38.5808333326384,63.6034202264699));
#126444=CARTESIAN_POINT('',(-13.0856980517762,39.1661587946801,63.2587206975987));
#126445=CARTESIAN_POINT('Ctrl Pts',(-13.0856980517762,39.1661587946801,
63.2587206975987));
#126446=CARTESIAN_POINT('Ctrl Pts',(-12.9106059326522,38.9910541747943,
63.3365689270392));
#126447=CARTESIAN_POINT('Ctrl Pts',(-12.6901619533851,38.8388876989633,
63.4261076675721));
#126448=CARTESIAN_POINT('Ctrl Pts',(-12.2008654839661,38.6335041042048,
63.5611995838646));
#126449=CARTESIAN_POINT('Ctrl Pts',(-11.9310804859103,38.5803311409929,
63.6034202264699));
#126450=CARTESIAN_POINT('Ctrl Pts',(-11.6715054007694,38.5803218750975,
63.6034202264699));
#126451=CARTESIAN_POINT('',(-13.9073268007583,39.9878462041285,63.0263984455991));
#126452=CARTESIAN_POINT('Origin',(-14.3044194064105,40.3849671603434,66.));
#126453=CARTESIAN_POINT('Ctrl Pts',(-13.9073268007584,39.9878462041285,
63.0263984455991));
#126454=CARTESIAN_POINT('Ctrl Pts',(-13.9960100566734,40.076535791615,63.0145549020595));
#126455=CARTESIAN_POINT('Ctrl Pts',(-14.0730534099154,40.1890412751135,
63.0038655192316));
#126456=CARTESIAN_POINT('Ctrl Pts',(-14.1339891648514,40.3361862550399,
63.0003015081353));
#126457=CARTESIAN_POINT('Ctrl Pts',(-14.1429487704599,40.3604431105938,
62.9999999999987));
#126458=CARTESIAN_POINT('Ctrl Pts',(-14.1509424007594,40.384961681931,63.));
#126459=CARTESIAN_POINT('Origin',(16.0005712344353,40.3838853813626,86.));
#126460=CARTESIAN_POINT('',(16.0005576038968,40.0020390449739,83.0244003328805));
#126461=CARTESIAN_POINT('',(16.0005576038968,40.0020390449739,88.9755996671195));
#126462=CARTESIAN_POINT('',(16.0005576038968,40.0020390450537,56.));
#126463=CARTESIAN_POINT('Origin',(16.0005712344353,40.3838853813626,86.));
#126464=CARTESIAN_POINT('Origin',(-25.9994287388058,40.3853846300409,86.));
#126465=CARTESIAN_POINT('',(-16.000205842957,40.3850276938095,83.));
#126466=CARTESIAN_POINT('Origin',(-16.000205842957,40.3850276938095,86.));
#126467=CARTESIAN_POINT('',(-14.1509424007594,40.3849616818491,83.));
#126468=CARTESIAN_POINT('',(-25.9994287388058,40.3853846300409,83.));
#126469=CARTESIAN_POINT('',(-14.2001947782207,40.6949634400972,83.0160596520708));
#126470=CARTESIAN_POINT('Ctrl Pts',(-14.1509424007594,40.384961681931,83.));
#126471=CARTESIAN_POINT('Ctrl Pts',(-14.1842343067511,40.4870767337193,
83.0000000000055));
#126472=CARTESIAN_POINT('Ctrl Pts',(-14.2001983851187,40.5939196884095,
83.0055622696198));
#126473=CARTESIAN_POINT('Ctrl Pts',(-14.2001947782208,40.6949634400972,
83.0160596520708));
#126474=CARTESIAN_POINT('',(-14.200125669996,42.6309634388637,84.0111601371654));
#126475=CARTESIAN_POINT('Origin',(-14.2002058441038,40.3849634402947,86.));
#126476=CARTESIAN_POINT('',(-13.700107822116,43.1309455903466,84.7919089438291));
#126477=CARTESIAN_POINT('Ctrl Pts',(-13.700107822116,43.1309455903466,84.7919089438292));
#126478=CARTESIAN_POINT('Ctrl Pts',(-13.7344681318913,43.1309468168859,
84.7919089438292));
#126479=CARTESIAN_POINT('Ctrl Pts',(-13.76624790509,43.1274886274743,84.7839956698363));
#126480=CARTESIAN_POINT('Ctrl Pts',(-13.8258360433629,43.1158302297232,
84.7580245352879));
#126481=CARTESIAN_POINT('Ctrl Pts',(-13.8536394068926,43.1076076153794,
84.739965262305));
#126482=CARTESIAN_POINT('Ctrl Pts',(-13.9314960885267,43.0776671514126,
84.6765650238703));
#126483=CARTESIAN_POINT('Ctrl Pts',(-13.9757656431352,43.0505415815266,
84.6222760175062));
#126484=CARTESIAN_POINT('Ctrl Pts',(-14.0695955559554,42.9760100922221,
84.4847585375541));
#126485=CARTESIAN_POINT('Ctrl Pts',(-14.1169980465718,42.9170084867485,
84.3867107678662));
#126486=CARTESIAN_POINT('Ctrl Pts',(-14.1825405634598,42.7822411369273,
84.1925083525136));
#126487=CARTESIAN_POINT('Ctrl Pts',(-14.2001229797765,42.7063273319006,
84.0962687007213));
#126488=CARTESIAN_POINT('Ctrl Pts',(-14.2001256699959,42.6309634388638,
84.0111601371654));
#126489=CARTESIAN_POINT('',(-12.8001078226894,43.1309134635892,84.7919089438291));
#126490=CARTESIAN_POINT('',(-25.9993307164994,43.1313846282914,84.7919089438291));
#126491=CARTESIAN_POINT('',(-12.8001078226894,43.1309134635892,87.2080910561709));
#126492=CARTESIAN_POINT('Ctrl Pts',(-12.8001078226893,43.1309134635892,
87.2080910561709));
#126493=CARTESIAN_POINT('Ctrl Pts',(-12.7874290218161,43.1309130110017,
87.2080910561709));
#126494=CARTESIAN_POINT('Ctrl Pts',(-12.7747450872089,43.1317310514822,
87.2062354373186));
#126495=CARTESIAN_POINT('Ctrl Pts',(-12.7501661862404,43.1348375455173,
87.199133868969));
#126496=CARTESIAN_POINT('Ctrl Pts',(-12.7382804382214,43.1371385398321,
87.193861533145));
#126497=CARTESIAN_POINT('Ctrl Pts',(-12.7046747516163,43.1455281504129,
87.1743800110828));
#126498=CARTESIAN_POINT('Ctrl Pts',(-12.6851453672407,43.1532658613644,
87.1561143770981));
#126499=CARTESIAN_POINT('Ctrl Pts',(-12.6471649980075,43.1716314784724,
87.1112980566841));
#126500=CARTESIAN_POINT('Ctrl Pts',(-12.6264424973877,43.1855881094717,
87.0757741121274));
#126501=CARTESIAN_POINT('Ctrl Pts',(-12.5778499600881,43.224674918756,86.9705448594992));
#126502=CARTESIAN_POINT('Ctrl Pts',(-12.5550921166024,43.2558293923731,
86.8746617707269));
#126503=CARTESIAN_POINT('Ctrl Pts',(-12.5029059493652,43.3441575831397,
86.5522053662921));
#126504=CARTESIAN_POINT('Ctrl Pts',(-12.5036463989442,43.3849028811464,
86.2522550206409));
#126505=CARTESIAN_POINT('Ctrl Pts',(-12.5036463989442,43.3849028811464,
85.7477449793591));
#126506=CARTESIAN_POINT('Ctrl Pts',(-12.5029059493652,43.3441575831397,
85.4477946337079));
#126507=CARTESIAN_POINT('Ctrl Pts',(-12.5550921166024,43.2558293923731,
85.1253382292731));
#126508=CARTESIAN_POINT('Ctrl Pts',(-12.5778499600881,43.224674918756,85.0294551405008));
#126509=CARTESIAN_POINT('Ctrl Pts',(-12.6264424973877,43.1855881094717,
84.9242258878726));
#126510=CARTESIAN_POINT('Ctrl Pts',(-12.6471649980075,43.1716314784724,
84.8887019433159));
#126511=CARTESIAN_POINT('Ctrl Pts',(-12.6851453672407,43.1532658613644,
84.8438856229019));
#126512=CARTESIAN_POINT('Ctrl Pts',(-12.7046747516163,43.1455281504129,
84.8256199889172));
#126513=CARTESIAN_POINT('Ctrl Pts',(-12.7382804382214,43.1371385398321,
84.806138466855));
#126514=CARTESIAN_POINT('Ctrl Pts',(-12.7501661862404,43.1348375455173,
84.800866131031));
#126515=CARTESIAN_POINT('Ctrl Pts',(-12.7747450872088,43.1317310514822,
84.7937645626813));
#126516=CARTESIAN_POINT('Ctrl Pts',(-12.7874290218161,43.1309130110017,
84.7919089438291));
#126517=CARTESIAN_POINT('Ctrl Pts',(-12.8001078226893,43.1309134635892,
84.7919089438291));
#126518=CARTESIAN_POINT('',(-13.700107822116,43.1309455903466,87.2080910561709));
#126519=CARTESIAN_POINT('',(-25.9993307164994,43.1313846282914,87.2080910561709));
#126520=CARTESIAN_POINT('',(-14.200125669996,42.6309634388637,87.9888398628346));
#126521=CARTESIAN_POINT('Ctrl Pts',(-14.2001256699959,42.6309634388638,
87.9888398628346));
#126522=CARTESIAN_POINT('Ctrl Pts',(-14.2001229797765,42.7063273319006,
87.9037312992787));
#126523=CARTESIAN_POINT('Ctrl Pts',(-14.1825405634598,42.7822411369273,
87.8074916474864));
#126524=CARTESIAN_POINT('Ctrl Pts',(-14.1169980465718,42.9170084867485,
87.6132892321338));
#126525=CARTESIAN_POINT('Ctrl Pts',(-14.0695955559553,42.9760100922221,
87.5152414624458));
#126526=CARTESIAN_POINT('Ctrl Pts',(-13.9757656431352,43.0505415815266,
87.3777239824938));
#126527=CARTESIAN_POINT('Ctrl Pts',(-13.9314960885267,43.0776671514126,
87.3234349761297));
#126528=CARTESIAN_POINT('Ctrl Pts',(-13.8536394068926,43.1076076153794,
87.260034737695));
#126529=CARTESIAN_POINT('Ctrl Pts',(-13.8258360433629,43.1158302297232,
87.2419754647121));
#126530=CARTESIAN_POINT('Ctrl Pts',(-13.76624790509,43.1274886274743,87.2160043301637));
#126531=CARTESIAN_POINT('Ctrl Pts',(-13.7344681318912,43.1309468168859,
87.2080910561708));
#126532=CARTESIAN_POINT('Ctrl Pts',(-13.700107822116,43.1309455903466,87.2080910561708));
#126533=CARTESIAN_POINT('',(-14.2001947782207,40.6949634400972,88.9839403479292));
#126534=CARTESIAN_POINT('Origin',(-14.2002058441038,40.3849634402947,86.));
#126535=CARTESIAN_POINT('',(-13.9073268007584,39.9878462041285,88.9736015544009));
#126536=CARTESIAN_POINT('Ctrl Pts',(-13.9073268007584,39.9878462041285,
88.9736015544009));
#126537=CARTESIAN_POINT('Ctrl Pts',(-13.9960100566734,40.076535791615,88.9854450979405));
#126538=CARTESIAN_POINT('Ctrl Pts',(-14.0730534099154,40.1890412751135,
88.9961344807684));
#126539=CARTESIAN_POINT('Ctrl Pts',(-14.1751560019799,40.435594122051,89.0021062582817));
#126540=CARTESIAN_POINT('Ctrl Pts',(-14.2001992511613,40.5696583440676,
88.9969582287394));
#126541=CARTESIAN_POINT('Ctrl Pts',(-14.2001947782208,40.6949634400972,
88.9839403479292));
#126542=CARTESIAN_POINT('',(-13.0856980517762,39.1661587946801,88.7412793024013));
#126543=CARTESIAN_POINT('Origin',(-14.3044194064105,40.3849671603434,86.));
#126544=CARTESIAN_POINT('',(-11.6715054007694,38.5803218750975,88.3965797735301));
#126545=CARTESIAN_POINT('Ctrl Pts',(-11.6715054007694,38.5803218750975,
88.3965797735301));
#126546=CARTESIAN_POINT('Ctrl Pts',(-11.9310804859103,38.5803311409929,
88.3965797735301));
#126547=CARTESIAN_POINT('Ctrl Pts',(-12.2008654839661,38.6335041042048,
88.4388004161354));
#126548=CARTESIAN_POINT('Ctrl Pts',(-12.6901619533851,38.8388876989633,
88.5738923324279));
#126549=CARTESIAN_POINT('Ctrl Pts',(-12.9106059326522,38.9910541747943,
88.6634310729608));
#126550=CARTESIAN_POINT('Ctrl Pts',(-13.0856980517762,39.1661587946801,
88.7412793024013));
#126551=CARTESIAN_POINT('',(-9.57050540210797,38.5802468769672,88.3965797735301));
#126552=CARTESIAN_POINT('',(-25.9994931547856,38.5808333326384,88.3965797735301));
#126553=CARTESIAN_POINT('',(-6.03491922226453,40.0445867642791,88.980661345019));
#126554=CARTESIAN_POINT('Ctrl Pts',(-6.03491922226454,40.0445867642791,
88.980661345019));
#126555=CARTESIAN_POINT('Ctrl Pts',(-6.46491979272286,39.6146168916673,
88.9316012220604));
#126556=CARTESIAN_POINT('Ctrl Pts',(-6.98352950944328,39.2568425175939,
88.7941482303742));
#126557=CARTESIAN_POINT('Ctrl Pts',(-8.18737580567769,38.7250267702563,
88.519101496493));
#126558=CARTESIAN_POINT('Ctrl Pts',(-8.88897256914252,38.5802225487005,
88.3965797735301));
#126559=CARTESIAN_POINT('Ctrl Pts',(-9.57050540210795,38.5802468769672,
88.3965797735301));
#126560=CARTESIAN_POINT('',(-4.31517414500253,41.7642090685172,88.6639647170472));
#126561=CARTESIAN_POINT('Origin',(-5.69482187817972,40.3846598287309,86.));
#126562=CARTESIAN_POINT('',(-4.88081081954212,43.1299146855279,87.2097174218851));
#126563=CARTESIAN_POINT('Ctrl Pts',(-4.88081081954212,43.1299146855279,
87.2097174218852));
#126564=CARTESIAN_POINT('Ctrl Pts',(-4.82482221472671,43.1299126869364,
87.2097174218852));
#126565=CARTESIAN_POINT('Ctrl Pts',(-4.77320031795729,43.1241916785181,
87.2228273668612));
#126566=CARTESIAN_POINT('Ctrl Pts',(-4.67621148812538,43.104869821818,87.2652368623582));
#126567=CARTESIAN_POINT('Ctrl Pts',(-4.63083615831867,43.0912259898174,
87.2944976062003));
#126568=CARTESIAN_POINT('Ctrl Pts',(-4.50299531310251,43.0409837535405,
87.3962229005734));
#126569=CARTESIAN_POINT('Ctrl Pts',(-4.42918588082232,42.9947395232464,
87.4819738279894));
#126570=CARTESIAN_POINT('Ctrl Pts',(-4.28473708613121,42.8747600616692,
87.6785381778342));
#126571=CARTESIAN_POINT('Ctrl Pts',(-4.21173521992967,42.7838888359609,
87.808410822416));
#126572=CARTESIAN_POINT('Ctrl Pts',(-4.10948896604543,42.5724250222423,
88.0592085197964));
#126573=CARTESIAN_POINT('Ctrl Pts',(-4.08083503287426,42.4515873535033,
88.1801672395615));
#126574=CARTESIAN_POINT('Ctrl Pts',(-4.08084269258333,42.2370080209205,
88.3629383226615));
#126575=CARTESIAN_POINT('Ctrl Pts',(-4.09805029004739,42.1312231898084,
88.4421976606013));
#126576=CARTESIAN_POINT('Ctrl Pts',(-4.17859647402362,41.9330114055893,
88.5720688356092));
#126577=CARTESIAN_POINT('Ctrl Pts',(-4.23902256544591,41.8403552115938,
88.6245291895113));
#126578=CARTESIAN_POINT('Ctrl Pts',(-4.31517414500254,41.7642090685172,
88.6639647170472));
#126579=CARTESIAN_POINT('',(-7.19981081806464,43.1299974654728,87.209717421885));
#126580=CARTESIAN_POINT('',(-25.9993307420611,43.1306685406019,87.2097174218847));
#126581=CARTESIAN_POINT('',(-7.19981081806464,43.1299974654728,84.790282578115));
#126582=CARTESIAN_POINT('Ctrl Pts',(-7.19981081806464,43.1299974654728,
84.7902825781149));
#126583=CARTESIAN_POINT('Ctrl Pts',(-7.21250680486427,43.1299979186738,
84.7902825781149));
#126584=CARTESIAN_POINT('Ctrl Pts',(-7.22520787530932,43.1308190809083,
84.7921402324463));
#126585=CARTESIAN_POINT('Ctrl Pts',(-7.24981968793656,43.1339357989149,
84.7992497365214));
#126586=CARTESIAN_POINT('Ctrl Pts',(-7.26172119707253,43.13624393064,84.8045280031556));
#126587=CARTESIAN_POINT('Ctrl Pts',(-7.29537069273696,43.1446590481209,
84.8240319462817));
#126588=CARTESIAN_POINT('Ctrl Pts',(-7.31492435500479,43.1524197100444,
84.8423192550511));
#126589=CARTESIAN_POINT('Ctrl Pts',(-7.35294574461562,43.1708382902919,
84.8871870557474));
#126590=CARTESIAN_POINT('Ctrl Pts',(-7.37368596111585,43.1848338692446,
84.922750254659));
#126591=CARTESIAN_POINT('Ctrl Pts',(-7.42230928437433,43.2240280671579,
85.0280938938583));
#126592=CARTESIAN_POINT('Ctrl Pts',(-7.44506219926236,43.2552667477377,
85.1240810706962));
#126593=CARTESIAN_POINT('Ctrl Pts',(-7.49721225591252,43.34385822923,85.4469741746507));
#126594=CARTESIAN_POINT('Ctrl Pts',(-7.49636431121142,43.3847241392164,
85.7473663615792));
#126595=CARTESIAN_POINT('Ctrl Pts',(-7.49636431121142,43.3847241392164,
86.2526336384208));
#126596=CARTESIAN_POINT('Ctrl Pts',(-7.49721225591251,43.34385822923,86.5530258253493));
#126597=CARTESIAN_POINT('Ctrl Pts',(-7.44506219926236,43.2552667477377,
86.8759189293038));
#126598=CARTESIAN_POINT('Ctrl Pts',(-7.42230928437433,43.2240280671579,
86.9719061061417));
#126599=CARTESIAN_POINT('Ctrl Pts',(-7.37368596111585,43.1848338692446,
87.0772497453409));
#126600=CARTESIAN_POINT('Ctrl Pts',(-7.35294574461562,43.1708382902919,
87.1128129442526));
#126601=CARTESIAN_POINT('Ctrl Pts',(-7.31492435500479,43.1524197100444,
87.1576807449489));
#126602=CARTESIAN_POINT('Ctrl Pts',(-7.29537069273696,43.1446590481209,
87.1759680537183));
#126603=CARTESIAN_POINT('Ctrl Pts',(-7.26172119707253,43.13624393064,87.1954719968443));
#126604=CARTESIAN_POINT('Ctrl Pts',(-7.24981968793656,43.1339357989149,
87.2007502634786));
#126605=CARTESIAN_POINT('Ctrl Pts',(-7.22520787530932,43.1308190809083,
87.2078597675537));
#126606=CARTESIAN_POINT('Ctrl Pts',(-7.21250680486427,43.1299979186738,
87.209717421885));
#126607=CARTESIAN_POINT('Ctrl Pts',(-7.19981081806464,43.1299974654728,
87.2097174218851));
#126608=CARTESIAN_POINT('',(-4.88081081954212,43.1299146855279,84.7902825781149));
#126609=CARTESIAN_POINT('',(-25.9993307420611,43.1306685406019,84.7902825781153));
#126610=CARTESIAN_POINT('',(-4.31517414500253,41.7642090685172,83.3360352829528));
#126611=CARTESIAN_POINT('Ctrl Pts',(-4.31517414500253,41.7642090685172,
83.3360352829528));
#126612=CARTESIAN_POINT('Ctrl Pts',(-4.23902256544589,41.8403552115938,
83.3754708104887));
#126613=CARTESIAN_POINT('Ctrl Pts',(-4.17859647402362,41.9330114055893,
83.4279311643908));
#126614=CARTESIAN_POINT('Ctrl Pts',(-4.09805029004739,42.1312231898084,
83.5578023393987));
#126615=CARTESIAN_POINT('Ctrl Pts',(-4.08084269258333,42.2370080209205,
83.6370616773385));
#126616=CARTESIAN_POINT('Ctrl Pts',(-4.08083503287426,42.4515873535033,
83.8198327604385));
#126617=CARTESIAN_POINT('Ctrl Pts',(-4.10948896604541,42.5724250222423,
83.9407914802035));
#126618=CARTESIAN_POINT('Ctrl Pts',(-4.21173521992965,42.7838888359608,
84.191589177584));
#126619=CARTESIAN_POINT('Ctrl Pts',(-4.28473708613121,42.8747600616692,
84.3214618221658));
#126620=CARTESIAN_POINT('Ctrl Pts',(-4.42918588082232,42.9947395232464,
84.5180261720106));
#126621=CARTESIAN_POINT('Ctrl Pts',(-4.50299531310251,43.0409837535405,
84.6037770994266));
#126622=CARTESIAN_POINT('Ctrl Pts',(-4.63083615831867,43.0912259898174,
84.7055023937997));
#126623=CARTESIAN_POINT('Ctrl Pts',(-4.67621148812538,43.104869821818,84.7347631376418));
#126624=CARTESIAN_POINT('Ctrl Pts',(-4.77320031795728,43.1241916785181,
84.7771726331388));
#126625=CARTESIAN_POINT('Ctrl Pts',(-4.82482221472671,43.1299126869364,
84.7902825781148));
#126626=CARTESIAN_POINT('Ctrl Pts',(-4.88081081954212,43.1299146855279,
84.7902825781148));
#126627=CARTESIAN_POINT('',(-5.69482187817968,40.384659828731,83.));
#126628=CARTESIAN_POINT('Origin',(-5.69482187817972,40.3846598287309,86.));
#126629=CARTESIAN_POINT('',(5.69537693071232,40.384253239671,83.));
#126630=CARTESIAN_POINT('',(-25.9994287388058,40.3853846300409,83.));
#126631=CARTESIAN_POINT('',(4.3155751451931,41.7640550251902,83.3361150636597));
#126632=CARTESIAN_POINT('Origin',(5.69537693071237,40.3842532396709,86.));
#126633=CARTESIAN_POINT('',(4.88126057014233,43.1297404501394,84.7906780580687));
#126634=CARTESIAN_POINT('Ctrl Pts',(4.88126057014233,43.1297404501394,84.7906780580686));
#126635=CARTESIAN_POINT('Ctrl Pts',(4.82527855129633,43.1297404501394,84.7906735213082));
#126636=CARTESIAN_POINT('Ctrl Pts',(4.77366641546815,43.1240229215084,84.7775580917314));
#126637=CARTESIAN_POINT('Ctrl Pts',(4.6766881693441,43.1047100794269,84.7351374178226));
#126638=CARTESIAN_POINT('Ctrl Pts',(4.63131473335929,43.0910704365374,84.7058682945448));
#126639=CARTESIAN_POINT('Ctrl Pts',(4.50347730469683,43.040841140764,84.6041166977585));
#126640=CARTESIAN_POINT('Ctrl Pts',(4.42966809762419,42.9946063244288,84.5183478507339));
#126641=CARTESIAN_POINT('Ctrl Pts',(4.28521059479939,42.8746430433406,84.3217402796909));
#126642=CARTESIAN_POINT('Ctrl Pts',(4.21219885970608,42.7837779689826,84.1918390912012));
#126643=CARTESIAN_POINT('Ctrl Pts',(4.10993073305515,42.5723177386494,83.9409875062198));
#126644=CARTESIAN_POINT('Ctrl Pts',(4.08126491520575,42.4514774729932,83.8200033709791));
#126645=CARTESIAN_POINT('Ctrl Pts',(4.08125725528774,42.2368922872938,83.6371990515189));
#126646=CARTESIAN_POINT('Ctrl Pts',(4.09845674449903,42.1311064778841,83.5579277928478));
#126647=CARTESIAN_POINT('Ctrl Pts',(4.17899207419104,41.9328803074183,83.4280312090116));
#126648=CARTESIAN_POINT('Ctrl Pts',(4.23941854432905,41.8402116260542,83.375558776258));
#126649=CARTESIAN_POINT('Ctrl Pts',(4.31557514519306,41.7640550251902,83.3361150636597));
#126650=CARTESIAN_POINT('',(7.20026057014233,43.1297404501395,84.7908660063353));
#126651=CARTESIAN_POINT('',(6.04076057014233,43.1297404501395,84.790772032202));
#126652=CARTESIAN_POINT('',(7.20026057014233,43.1297404501395,87.2091339936647));
#126653=CARTESIAN_POINT('Ctrl Pts',(7.20026057014233,43.1297404501395,87.2091339936647));
#126654=CARTESIAN_POINT('Ctrl Pts',(7.21294682501949,43.1297404501395,87.2091329653849));
#126655=CARTESIAN_POINT('Ctrl Pts',(7.22563810372133,43.1305598955788,87.2072760701667));
#126656=CARTESIAN_POINT('Ctrl Pts',(7.25023479260245,43.1336713801016,87.2001704115751));
#126657=CARTESIAN_POINT('Ctrl Pts',(7.2621307534533,43.1359764055222,87.1948942718855));
#126658=CARTESIAN_POINT('Ctrl Pts',(7.29576491915057,43.144380828481,87.1753983698309));
#126659=CARTESIAN_POINT('Ctrl Pts',(7.31531022822448,43.152132358212,87.1571188348341));
#126660=CARTESIAN_POINT('Ctrl Pts',(7.35331775020091,43.1705301900497,87.1122694969576));
#126661=CARTESIAN_POINT('Ctrl Pts',(7.3740522567382,43.1845108420159,87.0767203752738));
#126662=CARTESIAN_POINT('Ctrl Pts',(7.4226663467744,43.2236642757062,86.9714177547316));
#126663=CARTESIAN_POINT('Ctrl Pts',(7.44542247694709,43.2548716957552,86.8754679026737));
#126664=CARTESIAN_POINT('Ctrl Pts',(7.49758960390303,43.3433662832606,86.5527314566462));
#126665=CARTESIAN_POINT('Ctrl Pts',(7.49678217092917,43.3841889379055,86.2524977920887));
#126666=CARTESIAN_POINT('Ctrl Pts',(7.49678217092917,43.3841889379055,85.7475022079113));
#126667=CARTESIAN_POINT('Ctrl Pts',(7.49758960390304,43.3433662832606,85.4472685433538));
#126668=CARTESIAN_POINT('Ctrl Pts',(7.4454224769471,43.2548716957552,85.1245320973263));
#126669=CARTESIAN_POINT('Ctrl Pts',(7.4226663467744,43.2236642757062,85.0285822452685));
#126670=CARTESIAN_POINT('Ctrl Pts',(7.3740522567382,43.1845108420159,84.9232796247263));
#126671=CARTESIAN_POINT('Ctrl Pts',(7.35331775020092,43.1705301900497,84.8877305030424));
#126672=CARTESIAN_POINT('Ctrl Pts',(7.31531022822448,43.152132358212,84.8428811651659));
#126673=CARTESIAN_POINT('Ctrl Pts',(7.29576491915058,43.144380828481,84.8246016301691));
#126674=CARTESIAN_POINT('Ctrl Pts',(7.2621307534533,43.1359764055222,84.8051057281145));
#126675=CARTESIAN_POINT('Ctrl Pts',(7.25023479260245,43.1336713801016,84.7998295884249));
#126676=CARTESIAN_POINT('Ctrl Pts',(7.22563810372133,43.1305598955788,84.7927239298333));
#126677=CARTESIAN_POINT('Ctrl Pts',(7.21294682501949,43.1297404501395,84.7908670346151));
#126678=CARTESIAN_POINT('Ctrl Pts',(7.20026057014233,43.1297404501395,84.7908660063353));
#126679=CARTESIAN_POINT('',(4.88126057014233,43.1297404501394,87.2093219419313));
#126680=CARTESIAN_POINT('',(6.04076057014233,43.1297404501395,87.209227967798));
#126681=CARTESIAN_POINT('',(4.3155751451931,41.7640550251902,88.6638849363403));
#126682=CARTESIAN_POINT('Ctrl Pts',(4.31557514519306,41.7640550251902,88.6638849363403));
#126683=CARTESIAN_POINT('Ctrl Pts',(4.23941854432905,41.8402116260542,88.624441223742));
#126684=CARTESIAN_POINT('Ctrl Pts',(4.17899207419104,41.9328803074183,88.5719687909884));
#126685=CARTESIAN_POINT('Ctrl Pts',(4.09845674449903,42.1311064778841,88.4420722071522));
#126686=CARTESIAN_POINT('Ctrl Pts',(4.08125725528774,42.2368922872938,88.3628009484811));
#126687=CARTESIAN_POINT('Ctrl Pts',(4.08126491520575,42.4514774729932,88.1799966290208));
#126688=CARTESIAN_POINT('Ctrl Pts',(4.10993073305515,42.5723177386494,88.0590124937802));
#126689=CARTESIAN_POINT('Ctrl Pts',(4.21219885970609,42.7837779689826,87.8081609087987));
#126690=CARTESIAN_POINT('Ctrl Pts',(4.28521059479939,42.8746430433406,87.6782597203091));
#126691=CARTESIAN_POINT('Ctrl Pts',(4.42966809762419,42.9946063244288,87.4816521492661));
#126692=CARTESIAN_POINT('Ctrl Pts',(4.50347730469683,43.040841140764,87.3958833022415));
#126693=CARTESIAN_POINT('Ctrl Pts',(4.63131473335929,43.0910704365374,87.2941317054552));
#126694=CARTESIAN_POINT('Ctrl Pts',(4.6766881693441,43.1047100794269,87.2648625821774));
#126695=CARTESIAN_POINT('Ctrl Pts',(4.77366641546814,43.1240229215084,87.2224419082686));
#126696=CARTESIAN_POINT('Ctrl Pts',(4.82527855129633,43.1297404501394,87.2093264786918));
#126697=CARTESIAN_POINT('Ctrl Pts',(4.88126057014233,43.1297404501394,87.2093219419314));
#126698=CARTESIAN_POINT('',(6.03525883703878,40.0443713333445,88.9806859172054));
#126699=CARTESIAN_POINT('Origin',(5.69537693071237,40.3842532396709,86.));
#126700=CARTESIAN_POINT('',(9.57079274297153,38.5799052392773,88.3968369781133));
#126701=CARTESIAN_POINT('Ctrl Pts',(9.57079274297153,38.5799052392773,88.3968369781133));
#126702=CARTESIAN_POINT('Ctrl Pts',(9.5707332488234,38.5799052392773,88.3968369765146));
#126703=CARTESIAN_POINT('Ctrl Pts',(9.57067375482821,38.5799052403392,88.3968369757153));
#126704=CARTESIAN_POINT('Ctrl Pts',(8.88909486927776,38.5799295702497,88.3968369757153));
#126705=CARTESIAN_POINT('Ctrl Pts',(8.1875100639932,38.724779883745,88.519320896401));
#126706=CARTESIAN_POINT('Ctrl Pts',(6.98374971135328,39.2566553618154,88.7942694455703));
#126707=CARTESIAN_POINT('Ctrl Pts',(6.46520448621751,39.6144256841658,88.9316635383852));
#126708=CARTESIAN_POINT('Ctrl Pts',(6.03525883703882,40.0443713333445,88.9806859172054));
#126709=CARTESIAN_POINT('',(11.6717927429715,38.5799052392773,88.3968934308243));
#126710=CARTESIAN_POINT('',(10.6212927429715,38.5799052392773,88.3968652044688));
#126711=CARTESIAN_POINT('',(13.0860063053446,39.1656916769042,88.7414869339534));
#126712=CARTESIAN_POINT('Ctrl Pts',(13.0860063053446,39.1656916769042,88.7414869339534));
#126713=CARTESIAN_POINT('Ctrl Pts',(12.9115776150688,38.9912629866284,88.663969269128));
#126714=CARTESIAN_POINT('Ctrl Pts',(12.6925492447761,38.8399015743528,88.5750351340623));
#126715=CARTESIAN_POINT('Ctrl Pts',(12.2039210685268,38.6336428861301,88.4395838913209));
#126716=CARTESIAN_POINT('Ctrl Pts',(11.9328135534399,38.5799052392773,88.3969004440812));
#126717=CARTESIAN_POINT('Ctrl Pts',(11.6717927429715,38.5799052392773,88.3968934308243));
#126718=CARTESIAN_POINT('',(13.9076643850834,39.987349756643,88.973667809827));
#126719=CARTESIAN_POINT('Origin',(14.3042605619825,40.383945933542,86.));
#126720=CARTESIAN_POINT('',(14.2005576038968,40.6944565378947,88.9838876432241));
#126721=CARTESIAN_POINT('Ctrl Pts',(14.2005576038968,40.6944565378295,88.9838876425972));
#126722=CARTESIAN_POINT('Ctrl Pts',(14.2005576038968,40.69444463897,88.9838888808067));
#126723=CARTESIAN_POINT('Ctrl Pts',(14.2005576036844,40.6944327401709,88.9838901189379));
#126724=CARTESIAN_POINT('Ctrl Pts',(14.2005531444961,40.5695128967916,88.996887916041));
#126725=CARTESIAN_POINT('Ctrl Pts',(14.1756575752172,40.4358460629751,89.0020722846323));
#126726=CARTESIAN_POINT('Ctrl Pts',(14.0741268986634,40.1899012740497,88.9962434199587));
#126727=CARTESIAN_POINT('Ctrl Pts',(13.9975074091711,40.0776069665203,88.9856559212044));
#126728=CARTESIAN_POINT('Ctrl Pts',(13.9087580506029,39.988444692808,88.9738136974119));
#126729=CARTESIAN_POINT('Ctrl Pts',(13.9082116449317,39.9878970164913,88.9737408027343));
#126730=CARTESIAN_POINT('Ctrl Pts',(13.9076643850834,39.987349756643,88.973667809827));
#126731=CARTESIAN_POINT('',(14.2005576038968,42.6304565378295,87.9882672716729));
#126732=CARTESIAN_POINT('Origin',(14.2005576038968,40.383949635364,86.));
#126733=CARTESIAN_POINT('',(13.7005576038968,43.1304565378295,87.206978825168));
#126734=CARTESIAN_POINT('Ctrl Pts',(13.7005576038968,43.1304565378295,87.206978825168));
#126735=CARTESIAN_POINT('Ctrl Pts',(13.7005635533611,43.1304565378295,87.2069788246847));
#126736=CARTESIAN_POINT('Ctrl Pts',(13.7005695027606,43.1304565377233,87.2069788244431));
#126737=CARTESIAN_POINT('Ctrl Pts',(13.7349434333177,43.1304553106978,87.2069788244431));
#126738=CARTESIAN_POINT('Ctrl Pts',(13.7667215268191,43.1269938687308,87.2149030662356));
#126739=CARTESIAN_POINT('Ctrl Pts',(13.8263020113281,43.1153320791706,87.240899990775));
#126740=CARTESIAN_POINT('Ctrl Pts',(13.8540993385831,43.1071092325231,87.2589741809338));
#126741=CARTESIAN_POINT('Ctrl Pts',(13.9319395673727,43.0771707831725,87.3224216534088));
#126742=CARTESIAN_POINT('Ctrl Pts',(13.9761986813102,43.0500508066361,87.3767434803275));
#126743=CARTESIAN_POINT('Ctrl Pts',(14.070024541769,42.9755247782782,87.5143570677025));
#126744=CARTESIAN_POINT('Ctrl Pts',(14.1174300227276,42.916521123884,87.6124763023577));
#126745=CARTESIAN_POINT('Ctrl Pts',(14.1829744042219,42.7817463851036,87.8068079086529));
#126746=CARTESIAN_POINT('Ctrl Pts',(14.2005576038968,42.7058286960662,87.9031056458045));
#126747=CARTESIAN_POINT('Ctrl Pts',(14.2005576038968,42.6304565378295,87.9882672716729));
#126748=CARTESIAN_POINT('',(12.8005576038968,43.1304565378295,87.2070519271956));
#126749=CARTESIAN_POINT('',(13.2505576038968,43.1304565378295,87.2070153761818));
#126750=CARTESIAN_POINT('',(12.8005576038968,43.1304565378295,84.7929480728044));
#126751=CARTESIAN_POINT('Ctrl Pts',(12.8005576038968,43.1304565378295,84.7929480728043));
#126752=CARTESIAN_POINT('Ctrl Pts',(12.8005540342567,43.1304565378295,84.7929480725144));
#126753=CARTESIAN_POINT('Ctrl Pts',(12.800550464617,43.1304565378932,84.7929480723695));
#126754=CARTESIAN_POINT('Ctrl Pts',(12.8005468949777,43.1304565380206,84.7929480723695));
#126755=CARTESIAN_POINT('Ctrl Pts',(12.7878790745653,43.1304569902162,84.7929480723695));
#126756=CARTESIAN_POINT('Ctrl Pts',(12.775206184161,43.1312745218071,84.7948023896051));
#126757=CARTESIAN_POINT('Ctrl Pts',(12.7506486750991,43.1343773655443,84.8018988837129));
#126758=CARTESIAN_POINT('Ctrl Pts',(12.738773266856,43.1366751949132,84.8071674273606));
#126759=CARTESIAN_POINT('Ctrl Pts',(12.7051965550664,43.1450524580709,84.826634614644));
#126760=CARTESIAN_POINT('Ctrl Pts',(12.6856835914487,43.1527778071505,84.8448863925531));
#126761=CARTESIAN_POINT('Ctrl Pts',(12.6477316006356,43.1711140657731,84.8896697992273));
#126762=CARTESIAN_POINT('Ctrl Pts',(12.6270220730305,43.1850482619964,84.9251686425469));
#126763=CARTESIAN_POINT('Ctrl Pts',(12.5784538537086,43.2240722091775,85.0303247407441));
#126764=CARTESIAN_POINT('Ctrl Pts',(12.5556965844494,43.2551755942419,85.126141257432));
#126765=CARTESIAN_POINT('Ctrl Pts',(12.5034979555493,43.3433419209884,85.4483186441275));
#126766=CARTESIAN_POINT('Ctrl Pts',(12.5041748497398,43.3840101920279,85.7479867774995));
#126767=CARTESIAN_POINT('Ctrl Pts',(12.5041748497398,43.3840101920279,86.2520132225005));
#126768=CARTESIAN_POINT('Ctrl Pts',(12.5034979555493,43.3433419209884,86.5516813558725));
#126769=CARTESIAN_POINT('Ctrl Pts',(12.5556965844494,43.2551755942419,86.8738587425681));
#126770=CARTESIAN_POINT('Ctrl Pts',(12.5784538537086,43.2240722091775,86.9696752592559));
#126771=CARTESIAN_POINT('Ctrl Pts',(12.6270220730305,43.1850482619964,87.0748313574531));
#126772=CARTESIAN_POINT('Ctrl Pts',(12.6477316006356,43.1711140657731,87.1103302007727));
#126773=CARTESIAN_POINT('Ctrl Pts',(12.6856835914487,43.1527778071505,87.1551136074469));
#126774=CARTESIAN_POINT('Ctrl Pts',(12.7051965550664,43.1450524580709,87.173365385356));
#126775=CARTESIAN_POINT('Ctrl Pts',(12.738773266856,43.1366751949132,87.1928325726394));
#126776=CARTESIAN_POINT('Ctrl Pts',(12.7506486750991,43.1343773655443,87.198101116287));
#126777=CARTESIAN_POINT('Ctrl Pts',(12.775206184161,43.1312745218071,87.2051976103948));
#126778=CARTESIAN_POINT('Ctrl Pts',(12.7878790745653,43.1304569902162,87.2070519276305));
#126779=CARTESIAN_POINT('Ctrl Pts',(12.800550464617,43.1304565378932,87.2070519276305));
#126780=CARTESIAN_POINT('Ctrl Pts',(12.8005540342567,43.1304565378295,87.2070519274856));
#126781=CARTESIAN_POINT('Ctrl Pts',(12.8005576038968,43.1304565378295,87.2070519271956));
#126782=CARTESIAN_POINT('',(13.7005576038968,43.1304565378295,84.793021174832));
#126783=CARTESIAN_POINT('',(13.2505576038968,43.1304565378295,84.7929846238182));
#126784=CARTESIAN_POINT('',(14.2005576038968,42.6304565378295,84.0117327283271));
#126785=CARTESIAN_POINT('Ctrl Pts',(14.2005576038968,42.6304565378295,84.0117327283271));
#126786=CARTESIAN_POINT('Ctrl Pts',(14.2005576038968,42.7058286960663,84.0968943541956));
#126787=CARTESIAN_POINT('Ctrl Pts',(14.1829744042219,42.7817463851036,84.1931920913471));
#126788=CARTESIAN_POINT('Ctrl Pts',(14.1174300227276,42.916521123884,84.3875236976423));
#126789=CARTESIAN_POINT('Ctrl Pts',(14.070024541769,42.9755247782782,84.4856429322975));
#126790=CARTESIAN_POINT('Ctrl Pts',(13.9761986813102,43.0500508066361,84.6232565196725));
#126791=CARTESIAN_POINT('Ctrl Pts',(13.9319395673727,43.0771707831725,84.6775783465912));
#126792=CARTESIAN_POINT('Ctrl Pts',(13.8540993385831,43.1071092325231,84.7410258190662));
#126793=CARTESIAN_POINT('Ctrl Pts',(13.8263020113281,43.1153320791706,84.759100009225));
#126794=CARTESIAN_POINT('Ctrl Pts',(13.7667215268191,43.1269938687308,84.7850969337644));
#126795=CARTESIAN_POINT('Ctrl Pts',(13.7349434333177,43.1304553106978,84.7930211755569));
#126796=CARTESIAN_POINT('Ctrl Pts',(13.7005695027606,43.1304565377233,84.7930211755569));
#126797=CARTESIAN_POINT('Ctrl Pts',(13.7005635533611,43.1304565378295,84.7930211753153));
#126798=CARTESIAN_POINT('Ctrl Pts',(13.7005576038968,43.1304565378295,84.793021174832));
#126799=CARTESIAN_POINT('',(14.2005576038968,40.6944565378948,83.0161123567759));
#126800=CARTESIAN_POINT('Origin',(14.2005576038968,40.383949635364,86.));
#126801=CARTESIAN_POINT('',(14.1511293052103,40.3839513998532,83.));
#126802=CARTESIAN_POINT('Ctrl Pts',(14.1511293052103,40.3839513999301,83.));
#126803=CARTESIAN_POINT('Ctrl Pts',(14.184533612433,40.4862144071147,83.0000000000052));
#126804=CARTESIAN_POINT('Ctrl Pts',(14.2005539915515,40.5932423327881,83.0055811103851));
#126805=CARTESIAN_POINT('Ctrl Pts',(14.2005576036844,40.6944327401709,83.0161098810621));
#126806=CARTESIAN_POINT('Ctrl Pts',(14.2005576038968,40.69444463897,83.0161111191933));
#126807=CARTESIAN_POINT('Ctrl Pts',(14.2005576038968,40.6944565378295,83.0161123574028));
#126808=CARTESIAN_POINT('',(16.0005576038968,40.3838853818492,82.9999999980886));
#126809=CARTESIAN_POINT('',(-25.9994287388058,40.3853846300409,83.));
#126810=CARTESIAN_POINT('Origin',(16.0005576038968,40.3838853818492,86.));
#126811=CARTESIAN_POINT('Origin',(16.0005576038968,40.3838853818492,86.));
#126812=CARTESIAN_POINT('',(13.9076643850834,39.987349756643,83.026332190173));
#126813=CARTESIAN_POINT('Ctrl Pts',(13.9076643850834,39.987349756643,83.0263321901729));
#126814=CARTESIAN_POINT('Ctrl Pts',(13.9082116449317,39.9878970164913,83.0262591972656));
#126815=CARTESIAN_POINT('Ctrl Pts',(13.9087580506029,39.988444692808,83.0261863025881));
#126816=CARTESIAN_POINT('Ctrl Pts',(13.9975074091711,40.0776069665203,83.0143440787956));
#126817=CARTESIAN_POINT('Ctrl Pts',(14.0741268986634,40.1899012740497,83.0037565800413));
#126818=CARTESIAN_POINT('Ctrl Pts',(14.1345364020809,40.3362353976012,83.000288477273));
#126819=CARTESIAN_POINT('Ctrl Pts',(14.1432949797111,40.3599676160584,82.9999999999988));
#126820=CARTESIAN_POINT('Ctrl Pts',(14.1511293052103,40.3839513999301,83.));
#126821=CARTESIAN_POINT('',(13.0860063053446,39.1656916769042,83.2585130660466));
#126822=CARTESIAN_POINT('Origin',(14.3042605619825,40.383945933542,86.));
#126823=CARTESIAN_POINT('',(11.6717927429715,38.5799052392773,83.6031065691756));
#126824=CARTESIAN_POINT('Ctrl Pts',(11.6717927429715,38.5799052392773,83.6031065691756));
#126825=CARTESIAN_POINT('Ctrl Pts',(11.9328135534399,38.5799052392773,83.6030995559188));
#126826=CARTESIAN_POINT('Ctrl Pts',(12.2039210685268,38.6336428861301,83.5604161086791));
#126827=CARTESIAN_POINT('Ctrl Pts',(12.6925492447761,38.8399015743528,83.4249648659377));
#126828=CARTESIAN_POINT('Ctrl Pts',(12.9115776150688,38.9912629866284,83.336030730872));
#126829=CARTESIAN_POINT('Ctrl Pts',(13.0860063053446,39.1656916769042,83.2585130660466));
#126830=CARTESIAN_POINT('',(9.57079274297153,38.5799052392773,83.6031630218867));
#126831=CARTESIAN_POINT('',(10.6212927429715,38.5799052392773,83.6031347955312));
#126832=CARTESIAN_POINT('',(6.03525883703878,40.0443713333445,83.0193140827946));
#126833=CARTESIAN_POINT('Ctrl Pts',(6.0352588370388,40.0443713333445,83.0193140827946));
#126834=CARTESIAN_POINT('Ctrl Pts',(6.4652044862175,39.6144256841658,83.0683364616148));
#126835=CARTESIAN_POINT('Ctrl Pts',(6.98374971135328,39.2566553618154,83.2057305544296));
#126836=CARTESIAN_POINT('Ctrl Pts',(8.1875100639932,38.724779883745,83.4806791035989));
#126837=CARTESIAN_POINT('Ctrl Pts',(8.88909486927776,38.5799295702497,83.6031630242847));
#126838=CARTESIAN_POINT('Ctrl Pts',(9.57061426098601,38.5799052424629,83.6031630242847));
#126839=CARTESIAN_POINT('Ctrl Pts',(9.57067375482821,38.5799052403392,83.6031630242847));
#126840=CARTESIAN_POINT('Ctrl Pts',(9.5707332488234,38.5799052392773,83.6031630234854));
#126841=CARTESIAN_POINT('Ctrl Pts',(9.57079274297153,38.5799052392773,83.6031630218867));
#126842=CARTESIAN_POINT('Origin',(5.69537693071237,40.3842532396709,86.));
#126843=CARTESIAN_POINT('',(-6.03491922226453,40.0445867642791,83.019338654981));
#126844=CARTESIAN_POINT('Origin',(-5.69482187817972,40.3846598287309,86.));
#126845=CARTESIAN_POINT('',(-9.57050540210797,38.5802468769672,83.6034202264699));
#126846=CARTESIAN_POINT('Ctrl Pts',(-9.57050540210795,38.5802468769672,
83.6034202264699));
#126847=CARTESIAN_POINT('Ctrl Pts',(-8.88897256914252,38.5802225487005,
83.6034202264699));
#126848=CARTESIAN_POINT('Ctrl Pts',(-8.18737580567768,38.7250267702563,
83.480898503507));
#126849=CARTESIAN_POINT('Ctrl Pts',(-6.98352950944328,39.2568425175939,
83.2058517696258));
#126850=CARTESIAN_POINT('Ctrl Pts',(-6.46491979272285,39.6146168916673,
83.0683987779395));
#126851=CARTESIAN_POINT('Ctrl Pts',(-6.03491922226454,40.0445867642791,
83.019338654981));
#126852=CARTESIAN_POINT('',(-11.6715054007694,38.5803218750975,83.6034202264699));
#126853=CARTESIAN_POINT('',(-25.9994931547856,38.5808333326384,83.6034202264699));
#126854=CARTESIAN_POINT('',(-13.0856980517762,39.1661587946801,83.2587206975987));
#126855=CARTESIAN_POINT('Ctrl Pts',(-13.0856980517762,39.1661587946801,
83.2587206975987));
#126856=CARTESIAN_POINT('Ctrl Pts',(-12.9106059326522,38.9910541747942,
83.3365689270392));
#126857=CARTESIAN_POINT('Ctrl Pts',(-12.6901619533851,38.8388876989633,
83.4261076675721));
#126858=CARTESIAN_POINT('Ctrl Pts',(-12.2008654839661,38.6335041042048,
83.5611995838646));
#126859=CARTESIAN_POINT('Ctrl Pts',(-11.9310804859103,38.5803311409929,
83.6034202264699));
#126860=CARTESIAN_POINT('Ctrl Pts',(-11.6715054007694,38.5803218750975,
83.6034202264699));
#126861=CARTESIAN_POINT('',(-13.9073268007584,39.9878462041285,83.0263984455991));
#126862=CARTESIAN_POINT('Origin',(-14.3044194064105,40.3849671603434,86.));
#126863=CARTESIAN_POINT('Ctrl Pts',(-13.9073268007584,39.9878462041285,
83.0263984455991));
#126864=CARTESIAN_POINT('Ctrl Pts',(-13.9960100566734,40.076535791615,83.0145549020595));
#126865=CARTESIAN_POINT('Ctrl Pts',(-14.0730534099154,40.1890412751135,
83.0038655192316));
#126866=CARTESIAN_POINT('Ctrl Pts',(-14.1339891648514,40.3361862550399,
83.0003015081353));
#126867=CARTESIAN_POINT('Ctrl Pts',(-14.1429487704599,40.3604431105938,
82.9999999999987));
#126868=CARTESIAN_POINT('Ctrl Pts',(-14.1509424007594,40.384961681931,83.));
#126869=CARTESIAN_POINT('Origin',(-12.8000971137702,43.4309134633981,26.));
#126870=CARTESIAN_POINT('',(-12.8001078226894,43.1309134635892,26.));
#126871=CARTESIAN_POINT('',(-12.8001078226894,43.1309134635892,26.));
#126872=CARTESIAN_POINT('',(-12.5000971139614,43.4309027544789,26.));
#126873=CARTESIAN_POINT('Origin',(-12.8000971137702,43.4309134633981,26.));
#126874=CARTESIAN_POINT('',(-12.5000971139614,43.4309027544789,106.));
#126875=CARTESIAN_POINT('',(-12.5000971139614,43.4309027544789,26.));
#126876=CARTESIAN_POINT('',(-12.8001078226894,43.1309134635892,106.));
#126877=CARTESIAN_POINT('Origin',(-12.8000971137702,43.4309134633981,106.));
#126878=CARTESIAN_POINT('',(-12.8001078226894,43.1309134635892,26.));
#126879=CARTESIAN_POINT('',(-12.8001078226894,43.1309134635892,26.));
#126880=CARTESIAN_POINT('',(-12.8001078226894,43.1309134635892,26.));
#126881=CARTESIAN_POINT('Origin',(-12.8001078226894,43.1309134635892,26.));
#126882=CARTESIAN_POINT('',(-13.700107822116,43.1309455903466,26.));
#126883=CARTESIAN_POINT('',(-13.700107822116,43.1309455903466,26.));
#126884=CARTESIAN_POINT('',(-12.8001078226894,43.1309134635892,26.));
#126885=CARTESIAN_POINT('Origin',(-12.8001078226894,43.1309134635892,26.));
#126886=CARTESIAN_POINT('',(-13.700107822116,43.1309455903466,106.));
#126887=CARTESIAN_POINT('',(-12.8001078226894,43.1309134635892,106.));
#126888=CARTESIAN_POINT('',(-13.700107822116,43.1309455903466,26.));
#126889=CARTESIAN_POINT('Origin',(-12.8001078226894,43.1309134635892,26.));
#126890=CARTESIAN_POINT('',(-13.700107822116,43.1309455903466,26.));
#126891=CARTESIAN_POINT('Origin',(-13.7001256703145,42.6309455906652,26.));
#126892=CARTESIAN_POINT('',(-14.200125669996,42.6309634388637,26.));
#126893=CARTESIAN_POINT('',(-14.200125669996,42.6309634388637,26.));
#126894=CARTESIAN_POINT('Origin',(-13.7001256703145,42.6309455906652,26.));
#126895=CARTESIAN_POINT('Origin',(-13.7001256703145,42.6309455906652,26.));
#126896=CARTESIAN_POINT('',(-14.200125669996,42.6309634388637,106.));
#126897=CARTESIAN_POINT('Origin',(-13.7001256703145,42.6309455906652,106.));
#126898=CARTESIAN_POINT('',(-14.200125669996,42.6309634388637,26.));
#126899=CARTESIAN_POINT('Origin',(-13.7001256703145,42.6309455906652,26.));
#126900=CARTESIAN_POINT('',(-14.200125669996,42.6309634388637,26.));
#126901=CARTESIAN_POINT('Origin',(-14.200125669996,42.6309634388637,26.));
#126902=CARTESIAN_POINT('',(-14.2001947782207,40.6949634400972,26.));
#126903=CARTESIAN_POINT('',(-14.2001947782207,40.6949634400972,26.));
#126904=CARTESIAN_POINT('',(-14.200125669996,42.6309634388637,26.));
#126905=CARTESIAN_POINT('Origin',(-14.200125669996,42.6309634388637,26.));
#126906=CARTESIAN_POINT('',(-14.2001947782207,40.6949634400972,106.));
#126907=CARTESIAN_POINT('',(-14.200125669996,42.6309634388637,106.));
#126908=CARTESIAN_POINT('',(-14.2001947782207,40.6949634400972,26.));
#126909=CARTESIAN_POINT('Origin',(-14.200125669996,42.6309634388637,26.));
#126910=CARTESIAN_POINT('',(-14.2001947782207,40.6949634400972,26.));
#126911=CARTESIAN_POINT('Origin',(-13.2001947788579,40.6949277437001,26.));
#126912=CARTESIAN_POINT('',(-13.9073268007584,39.9878462041285,26.));
#126913=CARTESIAN_POINT('',(-13.9073268007584,39.9878462041285,26.));
#126914=CARTESIAN_POINT('Origin',(-13.2001947788579,40.6949277437001,26.));
#126915=CARTESIAN_POINT('Origin',(-13.2001947788579,40.6949277437001,26.));
#126916=CARTESIAN_POINT('',(-13.9073268007584,39.9878462041285,106.));
#126917=CARTESIAN_POINT('Origin',(-13.2001947788579,40.6949277437001,106.));
#126918=CARTESIAN_POINT('',(-13.9073268007584,39.9878462041285,26.));
#126919=CARTESIAN_POINT('Origin',(-13.2001947788579,40.6949277437001,26.));
#126920=CARTESIAN_POINT('',(-13.9073268007584,39.9878462041285,26.));
#126921=CARTESIAN_POINT('Origin',(-13.9073268007584,39.9878462041285,26.));
#126922=CARTESIAN_POINT('',(-13.0856980517762,39.1661587946801,26.));
#126923=CARTESIAN_POINT('',(-13.0856980517762,39.1661587946801,26.));
#126924=CARTESIAN_POINT('',(-13.9073268007584,39.9878462041285,26.));
#126925=CARTESIAN_POINT('Origin',(-13.9073268007584,39.9878462041285,26.));
#126926=CARTESIAN_POINT('',(-13.0856980517762,39.1661587946801,106.));
#126927=CARTESIAN_POINT('',(-13.9073268007584,39.9878462041285,106.));
#126928=CARTESIAN_POINT('',(-13.0856980517762,39.1661587946801,26.));
#126929=CARTESIAN_POINT('Origin',(-13.9073268007584,39.9878462041285,26.));
#126930=CARTESIAN_POINT('',(-13.0856980517762,39.1661587946801,26.));
#126931=CARTESIAN_POINT('Origin',(-11.6714340079752,40.5803218738233,26.));
#126932=CARTESIAN_POINT('',(-11.6715054007694,38.5803218750975,26.));
#126933=CARTESIAN_POINT('',(-11.6715054007694,38.5803218750975,26.));
#126934=CARTESIAN_POINT('Origin',(-11.6714340079752,40.5803218738233,26.));
#126935=CARTESIAN_POINT('Origin',(-11.6714340079752,40.5803218738233,26.));
#126936=CARTESIAN_POINT('',(-11.6715054007694,38.5803218750975,106.));
#126937=CARTESIAN_POINT('Origin',(-11.6714340079752,40.5803218738233,106.));
#126938=CARTESIAN_POINT('',(-11.6715054007694,38.5803218750975,26.));
#126939=CARTESIAN_POINT('Origin',(-11.6714340079752,40.5803218738233,26.));
#126940=CARTESIAN_POINT('',(-11.6715054007694,38.5803218750975,26.));
#126941=CARTESIAN_POINT('Origin',(-11.6715054007694,38.5803218750975,26.));
#126942=CARTESIAN_POINT('',(-9.57050540210797,38.5802468769672,26.));
#126943=CARTESIAN_POINT('',(-9.57050540210797,38.5802468769672,26.));
#126944=CARTESIAN_POINT('',(-11.6715054007694,38.5803218750975,26.));
#126945=CARTESIAN_POINT('Origin',(-11.6715054007694,38.5803218750975,26.));
#126946=CARTESIAN_POINT('',(-9.57050540210797,38.5802468769672,106.));
#126947=CARTESIAN_POINT('',(-11.6715054007694,38.5803218750975,106.));
#126948=CARTESIAN_POINT('',(-9.57050540210797,38.5802468769672,26.));
#126949=CARTESIAN_POINT('Origin',(-11.6715054007694,38.5803218750975,26.));
#126950=CARTESIAN_POINT('',(-9.57050540210797,38.5802468769672,26.));
#126951=CARTESIAN_POINT('Origin',(-9.57032692012244,43.5802468737816,26.));
#126952=CARTESIAN_POINT('',(-6.03491922226454,40.0445867642791,26.));
#126953=CARTESIAN_POINT('',(-6.03491922226454,40.0445867642791,26.));
#126954=CARTESIAN_POINT('Origin',(-9.57032692012244,43.5802468737816,26.));
#126955=CARTESIAN_POINT('Origin',(-9.57032692012244,43.5802468737816,26.));
#126956=CARTESIAN_POINT('',(-6.03491922226454,40.0445867642791,106.));
#126957=CARTESIAN_POINT('Origin',(-9.57032692012244,43.5802468737816,106.));
#126958=CARTESIAN_POINT('',(-6.03491922226454,40.0445867642791,26.));
#126959=CARTESIAN_POINT('Origin',(-9.57032692012244,43.5802468737816,26.));
#126960=CARTESIAN_POINT('',(-6.03491922226454,40.0445867642791,26.));
#126961=CARTESIAN_POINT('Origin',(-6.03491922226454,40.0445867642791,26.));
#126962=CARTESIAN_POINT('',(-4.31517414500253,41.7642090685172,26.));
#126963=CARTESIAN_POINT('',(-4.31517414500253,41.7642090685172,26.));
#126964=CARTESIAN_POINT('',(-6.03491922226454,40.0445867642791,26.));
#126965=CARTESIAN_POINT('Origin',(-6.03491922226454,40.0445867642791,26.));
#126966=CARTESIAN_POINT('',(-4.31517414500253,41.7642090685172,106.));
#126967=CARTESIAN_POINT('',(-6.03491922226454,40.0445867642791,106.));
#126968=CARTESIAN_POINT('',(-4.31517414500253,41.7642090685172,26.));
#126969=CARTESIAN_POINT('Origin',(-6.03491922226454,40.0445867642791,26.));
#126970=CARTESIAN_POINT('',(-4.31517414500253,41.7642090685172,26.));
#126971=CARTESIAN_POINT('Origin',(-4.8808393766598,42.3299146860376,26.));
#126972=CARTESIAN_POINT('',(-4.88081081954211,43.1299146855279,26.));
#126973=CARTESIAN_POINT('',(-4.88081081954211,43.1299146855279,26.));
#126974=CARTESIAN_POINT('Origin',(-4.8808393766598,42.3299146860376,26.));
#126975=CARTESIAN_POINT('Origin',(-4.8808393766598,42.3299146860376,26.));
#126976=CARTESIAN_POINT('',(-4.88081081954212,43.1299146855279,106.));
#126977=CARTESIAN_POINT('Origin',(-4.8808393766598,42.3299146860376,106.));
#126978=CARTESIAN_POINT('',(-4.88081081954211,43.1299146855279,26.));
#126979=CARTESIAN_POINT('Origin',(-4.8808393766598,42.3299146860376,26.));
#126980=CARTESIAN_POINT('',(-4.88081081954211,43.1299146855279,26.));
#126981=CARTESIAN_POINT('Origin',(-4.88081081954211,43.1299146855279,26.));
#126982=CARTESIAN_POINT('',(-7.19981081806464,43.1299974654728,26.));
#126983=CARTESIAN_POINT('',(-7.19981081806464,43.1299974654728,26.));
#126984=CARTESIAN_POINT('',(-4.88081081954211,43.1299146855279,26.));
#126985=CARTESIAN_POINT('Origin',(-4.88081081954211,43.1299146855279,26.));
#126986=CARTESIAN_POINT('',(-7.19981081806464,43.1299974654728,106.));
#126987=CARTESIAN_POINT('',(-4.88081081954211,43.1299146855279,106.));
#126988=CARTESIAN_POINT('',(-7.19981081806464,43.1299974654728,26.));
#126989=CARTESIAN_POINT('Origin',(-4.88081081954211,43.1299146855279,26.));
#126990=CARTESIAN_POINT('',(-7.19981081806464,43.1299974654728,26.));
#126991=CARTESIAN_POINT('Origin',(12.8005576038968,43.4304565378295,26.));
#126992=CARTESIAN_POINT('',(12.8005576038968,43.1304565378295,26.));
#126993=CARTESIAN_POINT('',(12.8005576038968,43.1304565378295,26.));
#126994=CARTESIAN_POINT('',(12.8005576038968,43.1304565378295,106.));
#126995=CARTESIAN_POINT('',(12.8005576038968,43.1304565378295,26.));
#126996=CARTESIAN_POINT('',(12.5005576038968,43.4304565378295,106.));
#126997=CARTESIAN_POINT('Origin',(12.8005576038968,43.4304565378295,106.));
#126998=CARTESIAN_POINT('',(12.5005576038968,43.4304565378295,26.));
#126999=CARTESIAN_POINT('',(12.5005576038968,43.4304565378295,26.));
#127000=CARTESIAN_POINT('',(12.8005576038968,43.1304565378295,26.));
#127001=CARTESIAN_POINT('Origin',(12.8005576038968,43.4304565378295,26.));
#127002=CARTESIAN_POINT('',(12.8005576038968,43.1304565378295,26.));
#127003=CARTESIAN_POINT('Origin',(12.8005576038968,43.1304565378295,26.));
#127004=CARTESIAN_POINT('',(13.7005576038968,43.1304565378295,106.));
#127005=CARTESIAN_POINT('',(13.7005576038968,43.1304565378295,26.));
#127006=CARTESIAN_POINT('',(12.8005576038968,43.1304565378295,106.));
#127007=CARTESIAN_POINT('Origin',(12.8005576038968,43.1304565378295,26.));
#127008=CARTESIAN_POINT('',(13.7005576038968,43.1304565378295,26.));
#127009=CARTESIAN_POINT('Origin',(12.8005576038968,43.1304565378295,26.));
#127010=CARTESIAN_POINT('',(13.7005576038968,43.1304565378295,26.));
#127011=CARTESIAN_POINT('Origin',(13.7005576038968,42.6304565378295,26.));
#127012=CARTESIAN_POINT('',(14.2005576038968,42.6304565378295,106.));
#127013=CARTESIAN_POINT('',(14.2005576038968,42.6304565378295,26.));
#127014=CARTESIAN_POINT('Origin',(13.7005576038968,42.6304565378295,106.));
#127015=CARTESIAN_POINT('Origin',(13.7005576038968,42.6304565378295,26.));
#127016=CARTESIAN_POINT('',(14.2005576038968,42.6304565378295,26.));
#127017=CARTESIAN_POINT('Origin',(13.7005576038968,42.6304565378295,26.));
#127018=CARTESIAN_POINT('',(14.2005576038968,42.6304565378295,26.));
#127019=CARTESIAN_POINT('Origin',(14.2005576038968,42.6304565378295,26.));
#127020=CARTESIAN_POINT('',(14.2005576038968,40.6944565378295,106.));
#127021=CARTESIAN_POINT('',(14.2005576038968,40.6944565378295,26.));
#127022=CARTESIAN_POINT('',(14.2005576038968,42.6304565378295,106.));
#127023=CARTESIAN_POINT('Origin',(14.2005576038968,42.6304565378295,26.));
#127024=CARTESIAN_POINT('',(14.2005576038968,40.6944565378295,26.));
#127025=CARTESIAN_POINT('Origin',(14.2005576038968,42.6304565378295,26.));
#127026=CARTESIAN_POINT('',(14.2005576038968,40.6944565378295,26.));
#127027=CARTESIAN_POINT('Origin',(13.2005576038968,40.6944565378295,26.));
#127028=CARTESIAN_POINT('',(13.9076643850834,39.987349756643,106.));
#127029=CARTESIAN_POINT('',(13.9076643850834,39.987349756643,26.));
#127030=CARTESIAN_POINT('Origin',(13.2005576038968,40.6944565378295,106.));
#127031=CARTESIAN_POINT('Origin',(13.2005576038968,40.6944565378295,26.));
#127032=CARTESIAN_POINT('',(13.9076643850834,39.987349756643,26.));
#127033=CARTESIAN_POINT('Origin',(13.2005576038968,40.6944565378295,26.));
#127034=CARTESIAN_POINT('',(13.9076643850834,39.987349756643,26.));
#127035=CARTESIAN_POINT('Origin',(13.9076643850834,39.987349756643,26.));
#127036=CARTESIAN_POINT('',(13.0860063053446,39.1656916769042,106.));
#127037=CARTESIAN_POINT('',(13.0860063053446,39.1656916769042,26.));
#127038=CARTESIAN_POINT('',(13.9076643850834,39.987349756643,106.));
#127039=CARTESIAN_POINT('Origin',(13.9076643850834,39.987349756643,26.));
#127040=CARTESIAN_POINT('',(13.0860063053446,39.1656916769042,26.));
#127041=CARTESIAN_POINT('Origin',(13.9076643850834,39.987349756643,26.));
#127042=CARTESIAN_POINT('',(13.0860063053446,39.1656916769042,26.));
#127043=CARTESIAN_POINT('Origin',(11.6717927429715,40.5799052392773,26.));
#127044=CARTESIAN_POINT('',(11.6717927429715,38.5799052392773,106.));
#127045=CARTESIAN_POINT('',(11.6717927429715,38.5799052392773,26.));
#127046=CARTESIAN_POINT('Origin',(11.6717927429715,40.5799052392773,106.));
#127047=CARTESIAN_POINT('Origin',(11.6717927429715,40.5799052392773,26.));
#127048=CARTESIAN_POINT('',(11.6717927429715,38.5799052392773,26.));
#127049=CARTESIAN_POINT('Origin',(11.6717927429715,40.5799052392773,26.));
#127050=CARTESIAN_POINT('',(11.6717927429715,38.5799052392773,26.));
#127051=CARTESIAN_POINT('Origin',(11.6717927429715,38.5799052392773,26.));
#127052=CARTESIAN_POINT('',(9.57079274297153,38.5799052392773,106.));
#127053=CARTESIAN_POINT('',(9.57079274297153,38.5799052392773,26.));
#127054=CARTESIAN_POINT('',(11.6717927429715,38.5799052392773,106.));
#127055=CARTESIAN_POINT('Origin',(11.6717927429715,38.5799052392773,26.));
#127056=CARTESIAN_POINT('',(9.57079274297153,38.5799052392773,26.));
#127057=CARTESIAN_POINT('Origin',(11.6717927429715,38.5799052392773,26.));
#127058=CARTESIAN_POINT('',(9.57079274297153,38.5799052392773,26.));
#127059=CARTESIAN_POINT('Origin',(9.57079274297151,43.5799052392773,26.));
#127060=CARTESIAN_POINT('',(6.03525883703878,40.0443713333445,106.));
#127061=CARTESIAN_POINT('',(6.03525883703878,40.0443713333445,26.));
#127062=CARTESIAN_POINT('Origin',(9.57079274297151,43.5799052392773,106.));
#127063=CARTESIAN_POINT('Origin',(9.57079274297151,43.5799052392773,26.));
#127064=CARTESIAN_POINT('',(6.03525883703878,40.0443713333445,26.));
#127065=CARTESIAN_POINT('Origin',(9.57079274297151,43.5799052392773,26.));
#127066=CARTESIAN_POINT('',(6.03525883703878,40.0443713333445,26.));
#127067=CARTESIAN_POINT('Origin',(6.03525883703878,40.0443713333445,26.));
#127068=CARTESIAN_POINT('',(4.31557514519309,41.7640550251902,106.));
#127069=CARTESIAN_POINT('',(4.31557514519309,41.7640550251902,26.));
#127070=CARTESIAN_POINT('',(6.03525883703878,40.0443713333445,106.));
#127071=CARTESIAN_POINT('Origin',(6.03525883703878,40.0443713333445,26.));
#127072=CARTESIAN_POINT('',(4.31557514519309,41.7640550251902,26.));
#127073=CARTESIAN_POINT('Origin',(6.03525883703878,40.0443713333445,26.));
#127074=CARTESIAN_POINT('',(4.31557514519309,41.7640550251902,26.));
#127075=CARTESIAN_POINT('Origin',(4.88126057014233,42.3297404501394,26.));
#127076=CARTESIAN_POINT('',(4.88126057014233,43.1297404501394,106.));
#127077=CARTESIAN_POINT('',(4.88126057014233,43.1297404501394,26.));
#127078=CARTESIAN_POINT('Origin',(4.88126057014233,42.3297404501394,106.));
#127079=CARTESIAN_POINT('Origin',(4.88126057014233,42.3297404501394,26.));
#127080=CARTESIAN_POINT('',(4.88126057014233,43.1297404501394,26.));
#127081=CARTESIAN_POINT('Origin',(4.88126057014233,42.3297404501394,26.));
#127082=CARTESIAN_POINT('',(4.88126057014233,43.1297404501394,26.));
#127083=CARTESIAN_POINT('Origin',(4.88126057014233,43.1297404501394,26.));
#127084=CARTESIAN_POINT('',(7.20026057014233,43.1297404501395,106.));
#127085=CARTESIAN_POINT('',(7.20026057014233,43.1297404501395,26.));
#127086=CARTESIAN_POINT('',(4.88126057014233,43.1297404501394,106.));
#127087=CARTESIAN_POINT('Origin',(4.88126057014233,43.1297404501394,26.));
#127088=CARTESIAN_POINT('',(7.20026057014233,43.1297404501395,26.));
#127089=CARTESIAN_POINT('Origin',(4.88126057014233,43.1297404501394,26.));
#127090=CARTESIAN_POINT('',(7.20026057014233,43.1297404501395,26.));
#127091=CARTESIAN_POINT('Origin',(-26.0001963416363,18.8817346167756,46.));
#127092=CARTESIAN_POINT('',(-26.0001963416363,18.8817346167756,43.5));
#127093=CARTESIAN_POINT('Origin',(-26.0001963416363,18.8817346167756,46.));
#127094=CARTESIAN_POINT('',(-19.0004228631993,18.8814847500817,43.5));
#127095=CARTESIAN_POINT('',(-26.0001963416363,18.8817346167756,43.5));
#127096=CARTESIAN_POINT('Origin',(-19.0004228631993,18.8814847500817,46.));
#127097=CARTESIAN_POINT('Origin',(-26.0001963416363,18.8817346167756,66.));
#127098=CARTESIAN_POINT('',(-26.0001963416363,18.8817346167756,63.5));
#127099=CARTESIAN_POINT('Origin',(-26.0001963416363,18.8817346167756,66.));
#127100=CARTESIAN_POINT('',(-19.0004228631993,18.8814847500817,63.5));
#127101=CARTESIAN_POINT('',(-26.0001963416363,18.8817346167756,63.5));
#127102=CARTESIAN_POINT('Origin',(-19.0004228631993,18.8814847500817,66.));
#127103=CARTESIAN_POINT('Origin',(-26.0001963416363,18.8817346167756,86.));
#127104=CARTESIAN_POINT('',(-26.0001963416363,18.8817346167756,83.5));
#127105=CARTESIAN_POINT('Origin',(-26.0001963416363,18.8817346167756,86.));
#127106=CARTESIAN_POINT('',(-19.0004228631993,18.8814847500817,83.5));
#127107=CARTESIAN_POINT('',(-26.0001963416363,18.8817346167756,83.5));
#127108=CARTESIAN_POINT('Origin',(-19.0004228631993,18.8814847500817,86.));
#127109=CARTESIAN_POINT('Origin',(0.,30.5305,26.));
#127110=CARTESIAN_POINT('',(-11.9999999923546,30.5309283567652,26.));
#127111=CARTESIAN_POINT('',(0.,30.5305,26.));
#127112=CARTESIAN_POINT('',(-11.9999999923546,30.5309283567652,26.));
#127113=CARTESIAN_POINT('',(0.,30.5305,106.));
#127114=CARTESIAN_POINT('',(0.,30.5305,26.));
#127115=CARTESIAN_POINT('',(-11.9999999923546,30.5309283567652,106.));
#127116=CARTESIAN_POINT('',(-11.9999999923546,30.5309283567652,106.));
#127117=CARTESIAN_POINT('',(-11.9999999923546,30.5309283567652,26.));
#127118=CARTESIAN_POINT('Origin',(-7.19973942527044,45.1299974641986,26.));
#127119=CARTESIAN_POINT('',(-7.19973942527044,45.1299974641986,26.));
#127120=CARTESIAN_POINT('',(-7.19973942527044,45.1299974641986,26.));
#127121=CARTESIAN_POINT('',(-7.19973942527044,45.1299974641986,106.));
#127122=CARTESIAN_POINT('',(-7.19973942527044,45.1299974641986,26.));
#127123=CARTESIAN_POINT('',(-7.19973942527044,45.1299974641986,106.));
#127124=CARTESIAN_POINT('Origin',(-7.19975013418957,44.8299974643897,26.));
#127125=CARTESIAN_POINT('',(-7.49975013399844,44.8300081733089,26.));
#127126=CARTESIAN_POINT('Origin',(-7.19975013418957,44.8299974643897,26.));
#127127=CARTESIAN_POINT('',(-7.49975013399844,44.8300081733089,106.));
#127128=CARTESIAN_POINT('',(-7.49975013399844,44.8300081733089,26.));
#127129=CARTESIAN_POINT('Origin',(-7.19975013418957,44.8299974643897,106.));
#127130=CARTESIAN_POINT('Origin',(-7.49980010895438,43.4300081742008,26.));
#127131=CARTESIAN_POINT('',(-7.49980010895438,43.4300081742008,26.));
#127132=CARTESIAN_POINT('',(-7.49980010895438,43.4300081742008,26.));
#127133=CARTESIAN_POINT('',(-7.49980010895438,43.4300081742008,106.));
#127134=CARTESIAN_POINT('',(-7.49980010895438,43.4300081742008,26.));
#127135=CARTESIAN_POINT('',(-7.49980010895438,43.4300081742008,106.));
#127136=CARTESIAN_POINT('Origin',(-7.19980010914551,43.4299974652817,26.));
#127137=CARTESIAN_POINT('',(-7.19981081806464,43.1299974654728,26.));
#127138=CARTESIAN_POINT('Origin',(-7.19980010914551,43.4299974652817,106.));
#127139=CARTESIAN_POINT('Origin',(-7.19980010914551,43.4299974652817,26.));
#127140=CARTESIAN_POINT('Origin',(-4.88081081954211,43.1299146855279,26.));
#127141=CARTESIAN_POINT('',(-4.88081081954211,43.1299146855279,26.));
#127142=CARTESIAN_POINT('Origin',(-4.8808393766598,42.3299146860376,26.));
#127143=CARTESIAN_POINT('',(-4.31517414500253,41.7642090685172,26.));
#127144=CARTESIAN_POINT('Origin',(-6.03491922226454,40.0445867642791,26.));
#127145=CARTESIAN_POINT('',(-6.03491922226454,40.0445867642791,26.));
#127146=CARTESIAN_POINT('Origin',(-9.57032692012244,43.5802468737816,26.));
#127147=CARTESIAN_POINT('',(-9.57050540210797,38.5802468769672,26.));
#127148=CARTESIAN_POINT('Origin',(-11.6715054007694,38.5803218750975,26.));
#127149=CARTESIAN_POINT('',(-11.6715054007694,38.5803218750975,26.));
#127150=CARTESIAN_POINT('Origin',(-11.6714340079752,40.5803218738233,26.));
#127151=CARTESIAN_POINT('',(-13.0856980517762,39.1661587946801,26.));
#127152=CARTESIAN_POINT('Origin',(-13.9073268007584,39.9878462041285,26.));
#127153=CARTESIAN_POINT('',(-13.9073268007584,39.9878462041285,26.));
#127154=CARTESIAN_POINT('Origin',(-13.2001947788579,40.6949277437001,26.));
#127155=CARTESIAN_POINT('',(-14.2001947782207,40.6949634400972,26.));
#127156=CARTESIAN_POINT('Origin',(-14.200125669996,42.6309634388637,26.));
#127157=CARTESIAN_POINT('',(-14.200125669996,42.6309634388637,26.));
#127158=CARTESIAN_POINT('Origin',(-13.7001256703145,42.6309455906652,26.));
#127159=CARTESIAN_POINT('',(-13.700107822116,43.1309455903466,26.));
#127160=CARTESIAN_POINT('Origin',(-12.8001078226894,43.1309134635892,26.));
#127161=CARTESIAN_POINT('Origin',(-12.5000471390054,44.830902753587,26.));
#127162=CARTESIAN_POINT('',(-12.5000471390054,44.830902753587,26.));
#127163=CARTESIAN_POINT('',(-12.5000471390054,44.830902753587,26.));
#127164=CARTESIAN_POINT('',(-12.5000471390054,44.830902753587,106.));
#127165=CARTESIAN_POINT('',(-12.5000471390054,44.830902753587,26.));
#127166=CARTESIAN_POINT('',(-12.5000471390054,44.830902753587,106.));
#127167=CARTESIAN_POINT('Origin',(-12.8000471388143,44.8309134625061,26.));
#127168=CARTESIAN_POINT('',(-12.8000364298952,45.130913462315,26.));
#127169=CARTESIAN_POINT('Origin',(-12.8000471388143,44.8309134625061,26.));
#127170=CARTESIAN_POINT('',(-12.8000364298952,45.130913462315,106.));
#127171=CARTESIAN_POINT('',(-12.8000364298952,45.130913462315,26.));
#127172=CARTESIAN_POINT('Origin',(-12.8000471388143,44.8309134625061,106.));
#127173=CARTESIAN_POINT('Origin',(-15.500036428175,45.1310098425871,26.));
#127174=CARTESIAN_POINT('',(-15.500036428175,45.1310098425871,26.));
#127175=CARTESIAN_POINT('',(-15.500036428175,45.1310098425871,26.));
#127176=CARTESIAN_POINT('',(-15.500036428175,45.1310098425871,106.));
#127177=CARTESIAN_POINT('',(-15.500036428175,45.1310098425871,26.));
#127178=CARTESIAN_POINT('',(-15.500036428175,45.1310098425871,106.));
#127179=CARTESIAN_POINT('Origin',(-15.5000542763735,44.6310098429057,26.));
#127180=CARTESIAN_POINT('',(-16.0000542760549,44.6310276911043,26.));
#127181=CARTESIAN_POINT('Origin',(-15.5000542763735,44.6310098429057,26.));
#127182=CARTESIAN_POINT('',(-16.0000542760549,44.6310276911043,106.));
#127183=CARTESIAN_POINT('',(-16.0000542760549,44.6310276911043,26.));
#127184=CARTESIAN_POINT('Origin',(-15.5000542763735,44.6310098429057,106.));
#127185=CARTESIAN_POINT('Origin',(-16.0003574098591,36.1390276965147,26.));
#127186=CARTESIAN_POINT('',(-16.0003574098591,36.1390276965147,26.));
#127187=CARTESIAN_POINT('',(-16.0003574098591,36.1390276965147,26.));
#127188=CARTESIAN_POINT('',(-16.0003574098591,36.1390276965147,106.));
#127189=CARTESIAN_POINT('',(-16.0003574098591,36.1390276965147,26.));
#127190=CARTESIAN_POINT('',(-16.0003574098591,36.1390276965147,106.));
#127191=CARTESIAN_POINT('Origin',(-16.5083574095355,36.1390458302844,26.));
#127192=CARTESIAN_POINT('',(-16.5083755433052,35.631045830608,26.));
#127193=CARTESIAN_POINT('Origin',(-16.5083574095355,36.1390458302844,26.));
#127194=CARTESIAN_POINT('',(-16.5083755433052,35.631045830608,106.));
#127195=CARTESIAN_POINT('',(-16.5083755433052,35.631045830608,26.));
#127196=CARTESIAN_POINT('Origin',(-16.5083574095355,36.1390458302844,106.));
#127197=CARTESIAN_POINT('Origin',(-16.8283755431013,35.6310572534551,26.));
#127198=CARTESIAN_POINT('',(-16.8283755431013,35.6310572534551,26.));
#127199=CARTESIAN_POINT('',(-16.8283755431013,35.6310572534551,26.));
#127200=CARTESIAN_POINT('',(-16.8283755431013,35.6310572534551,106.));
#127201=CARTESIAN_POINT('',(-16.8283755431013,35.6310572534551,26.));
#127202=CARTESIAN_POINT('',(-16.8283755431013,35.6310572534551,106.));
#127203=CARTESIAN_POINT('Origin',(-16.8284826322926,32.6310572553665,26.));
#127204=CARTESIAN_POINT('',(-18.9497272510074,34.7524533210679,26.));
#127205=CARTESIAN_POINT('Origin',(-16.8284826322926,32.6310572553665,26.));
#127206=CARTESIAN_POINT('',(-18.9497272510074,34.7524533210679,106.));
#127207=CARTESIAN_POINT('',(-18.9497272510074,34.7524533210679,26.));
#127208=CARTESIAN_POINT('Origin',(-16.8284826322926,32.6310572553665,106.));
#127209=CARTESIAN_POINT('Origin',(-24.5353630919994,29.167216239992,26.));
#127210=CARTESIAN_POINT('',(-24.5353630919994,29.167216239992,26.));
#127211=CARTESIAN_POINT('',(-24.5353630919994,29.167216239992,26.));
#127212=CARTESIAN_POINT('',(-24.5353630919994,29.167216239992,106.));
#127213=CARTESIAN_POINT('',(-24.5353630919994,29.167216239992,26.));
#127214=CARTESIAN_POINT('',(-24.5353630919994,29.167216239992,106.));
#127215=CARTESIAN_POINT('Origin',(-20.9999553941414,25.6315561304895,26.));
#127216=CARTESIAN_POINT('',(-25.9999553909559,25.631734612475,26.));
#127217=CARTESIAN_POINT('Origin',(-20.9999553941414,25.6315561304895,26.));
#127218=CARTESIAN_POINT('',(-25.9999553909559,25.631734612475,106.));
#127219=CARTESIAN_POINT('',(-25.9999553909559,25.631734612475,26.));
#127220=CARTESIAN_POINT('Origin',(-20.9999553941414,25.6315561304895,106.));
#127221=CARTESIAN_POINT('Origin',(-26.0004372923167,12.1317346210761,26.));
#127222=CARTESIAN_POINT('',(-26.0004372923167,12.1317346210761,26.));
#127223=CARTESIAN_POINT('',(-26.0004372923167,12.1317346210761,26.));
#127224=CARTESIAN_POINT('',(-26.0004372923167,12.1317346210761,106.));
#127225=CARTESIAN_POINT('',(-26.0004372923167,12.1317346210761,26.));
#127226=CARTESIAN_POINT('',(-26.0004372923167,12.1317346210761,106.));
#127227=CARTESIAN_POINT('Origin',(-25.0004372929538,12.131698924679,26.));
#127228=CARTESIAN_POINT('',(-25.0004729893509,11.1316989253161,26.));
#127229=CARTESIAN_POINT('Origin',(-25.0004372929538,12.131698924679,26.));
#127230=CARTESIAN_POINT('',(-25.0004729893509,11.1316989253161,106.));
#127231=CARTESIAN_POINT('',(-25.0004729893509,11.1316989253161,26.));
#127232=CARTESIAN_POINT('Origin',(-25.0004372929538,12.131698924679,106.));
#127233=CARTESIAN_POINT('Origin',(-20.500472992218,11.1315382915292,26.));
#127234=CARTESIAN_POINT('',(-20.500472992218,11.1315382915292,26.));
#127235=CARTESIAN_POINT('',(-20.500472992218,11.1315382915292,26.));
#127236=CARTESIAN_POINT('',(-20.500472992218,11.1315382915292,106.));
#127237=CARTESIAN_POINT('',(-20.500472992218,11.1315382915292,26.));
#127238=CARTESIAN_POINT('',(-20.500472992218,11.1315382915292,106.));
#127239=CARTESIAN_POINT('Origin',(-19.000645973767,12.6312582369605,26.));
#127240=CARTESIAN_POINT('',(-19.000645973767,12.6312582369605,26.));
#127241=CARTESIAN_POINT('',(-19.000645973767,12.6312582369605,26.));
#127242=CARTESIAN_POINT('',(-19.000645973767,12.6312582369605,106.));
#127243=CARTESIAN_POINT('',(-19.000645973767,12.6312582369605,26.));
#127244=CARTESIAN_POINT('',(-19.000645973767,12.6312582369605,106.));
#127245=CARTESIAN_POINT('Origin',(-19.0003186021092,21.8022582311175,26.));
#127246=CARTESIAN_POINT('',(-19.0003186021092,21.8022582311175,26.));
#127247=CARTESIAN_POINT('',(-19.0003186021092,21.8022582311175,26.));
#127248=CARTESIAN_POINT('',(-19.0003186021092,21.8022582311175,106.));
#127249=CARTESIAN_POINT('',(-19.0003186021092,21.8022582311175,26.));
#127250=CARTESIAN_POINT('',(-19.0003186021092,21.8022582311175,106.));
#127251=CARTESIAN_POINT('Origin',(-18.0003186027463,21.8022225347204,26.));
#127252=CARTESIAN_POINT('',(-18.4697586471852,22.6851868854601,26.));
#127253=CARTESIAN_POINT('Origin',(-18.0003186027463,21.8022225347204,26.));
#127254=CARTESIAN_POINT('',(-18.4697586471852,22.6851868854601,106.));
#127255=CARTESIAN_POINT('',(-18.4697586471852,22.6851868854601,26.));
#127256=CARTESIAN_POINT('Origin',(-18.0003186027463,21.8022225347204,106.));
#127257=CARTESIAN_POINT('Origin',(-15.7502284469069,24.1310622223319,26.));
#127258=CARTESIAN_POINT('',(-15.7502284469069,24.1310622223319,26.));
#127259=CARTESIAN_POINT('',(-15.7502284469069,24.1310622223319,26.));
#127260=CARTESIAN_POINT('',(-15.7502284469069,24.1310622223319,106.));
#127261=CARTESIAN_POINT('',(-15.7502284469069,24.1310622223319,26.));
#127262=CARTESIAN_POINT('',(-15.7502284469069,24.1310622223319,106.));
#127263=CARTESIAN_POINT('Origin',(-12.0002284492961,24.1309283608428,26.));
#127264=CARTESIAN_POINT('',(-12.0002284492961,24.1309283608428,26.));
#127265=CARTESIAN_POINT('',(-12.0002284492961,24.1309283608428,26.));
#127266=CARTESIAN_POINT('',(-12.0002284492961,24.1309283608428,106.));
#127267=CARTESIAN_POINT('',(-12.0002284492961,24.1309283608428,26.));
#127268=CARTESIAN_POINT('',(-12.0002284492961,24.1309283608428,106.));
#127269=CARTESIAN_POINT('Origin',(-11.9999999923546,30.5309283567652,26.));
#127270=CARTESIAN_POINT('',(-11.9999999923546,30.5309283567652,26.));
#127271=CARTESIAN_POINT('',(-11.9999999923546,30.5309283567652,106.));
#127272=CARTESIAN_POINT('Origin',(0.,30.5305,26.));
#127273=CARTESIAN_POINT('',(12.,30.5305,26.));
#127274=CARTESIAN_POINT('',(12.,30.5305,26.));
#127275=CARTESIAN_POINT('',(12.,30.5305,106.));
#127276=CARTESIAN_POINT('',(12.,30.5305,26.));
#127277=CARTESIAN_POINT('',(12.,30.5305,106.));
#127278=CARTESIAN_POINT('Origin',(7.20026057014233,44.8297404501395,26.));
#127279=CARTESIAN_POINT('',(7.50026057014233,44.8297404501395,26.));
#127280=CARTESIAN_POINT('Origin',(7.20026057014233,44.8297404501395,26.));
#127281=CARTESIAN_POINT('',(7.50026057014233,44.8297404501395,106.));
#127282=CARTESIAN_POINT('Origin',(7.20026057014233,44.8297404501395,106.));
#127283=CARTESIAN_POINT('',(7.50026057014233,44.8297404501395,26.));
#127284=CARTESIAN_POINT('Origin',(7.50026057014233,43.4297404501395,26.));
#127285=CARTESIAN_POINT('',(7.50026057014233,43.4297404501395,26.));
#127286=CARTESIAN_POINT('',(7.50026057014233,43.4297404501395,26.));
#127287=CARTESIAN_POINT('',(7.50026057014233,43.4297404501395,106.));
#127288=CARTESIAN_POINT('',(7.50026057014233,43.4297404501395,106.));
#127289=CARTESIAN_POINT('',(7.50026057014233,43.4297404501395,26.));
#127290=CARTESIAN_POINT('Origin',(7.20026057014232,43.4297404501395,26.));
#127291=CARTESIAN_POINT('',(7.20026057014233,43.1297404501395,26.));
#127292=CARTESIAN_POINT('',(7.20026057014233,43.1297404501395,26.));
#127293=CARTESIAN_POINT('Origin',(7.20026057014232,43.4297404501395,26.));
#127294=CARTESIAN_POINT('Origin',(7.20026057014232,43.4297404501395,106.));
#127295=CARTESIAN_POINT('Origin',(4.88126057014233,43.1297404501394,26.));
#127296=CARTESIAN_POINT('',(4.88126057014233,43.1297404501394,26.));
#127297=CARTESIAN_POINT('',(4.88126057014233,43.1297404501394,26.));
#127298=CARTESIAN_POINT('',(4.88126057014233,43.1297404501394,26.));
#127299=CARTESIAN_POINT('Origin',(4.88126057014233,42.3297404501394,26.));
#127300=CARTESIAN_POINT('',(4.31557514519309,41.7640550251902,26.));
#127301=CARTESIAN_POINT('',(4.31557514519309,41.7640550251902,26.));
#127302=CARTESIAN_POINT('Origin',(4.88126057014233,42.3297404501394,26.));
#127303=CARTESIAN_POINT('Origin',(6.03525883703878,40.0443713333445,26.));
#127304=CARTESIAN_POINT('',(6.03525883703878,40.0443713333445,26.));
#127305=CARTESIAN_POINT('',(6.03525883703878,40.0443713333445,26.));
#127306=CARTESIAN_POINT('',(6.03525883703878,40.0443713333445,26.));
#127307=CARTESIAN_POINT('Origin',(9.57079274297151,43.5799052392773,26.));
#127308=CARTESIAN_POINT('',(9.57079274297153,38.5799052392773,26.));
#127309=CARTESIAN_POINT('',(9.57079274297153,38.5799052392773,26.));
#127310=CARTESIAN_POINT('Origin',(9.57079274297151,43.5799052392773,26.));
#127311=CARTESIAN_POINT('Origin',(11.6717927429715,38.5799052392773,26.));
#127312=CARTESIAN_POINT('',(11.6717927429715,38.5799052392773,26.));
#127313=CARTESIAN_POINT('',(11.6717927429715,38.5799052392773,26.));
#127314=CARTESIAN_POINT('',(11.6717927429715,38.5799052392773,26.));
#127315=CARTESIAN_POINT('Origin',(11.6717927429715,40.5799052392773,26.));
#127316=CARTESIAN_POINT('',(13.0860063053446,39.1656916769042,26.));
#127317=CARTESIAN_POINT('',(13.0860063053446,39.1656916769042,26.));
#127318=CARTESIAN_POINT('Origin',(11.6717927429715,40.5799052392773,26.));
#127319=CARTESIAN_POINT('Origin',(13.9076643850834,39.987349756643,26.));
#127320=CARTESIAN_POINT('',(13.9076643850834,39.987349756643,26.));
#127321=CARTESIAN_POINT('',(13.9076643850834,39.987349756643,26.));
#127322=CARTESIAN_POINT('',(13.9076643850834,39.987349756643,26.));
#127323=CARTESIAN_POINT('Origin',(13.2005576038968,40.6944565378295,26.));
#127324=CARTESIAN_POINT('',(14.2005576038968,40.6944565378295,26.));
#127325=CARTESIAN_POINT('',(14.2005576038968,40.6944565378295,26.));
#127326=CARTESIAN_POINT('Origin',(13.2005576038968,40.6944565378295,26.));
#127327=CARTESIAN_POINT('Origin',(14.2005576038968,42.6304565378295,26.));
#127328=CARTESIAN_POINT('',(14.2005576038968,42.6304565378295,26.));
#127329=CARTESIAN_POINT('',(14.2005576038968,42.6304565378295,26.));
#127330=CARTESIAN_POINT('',(14.2005576038968,42.6304565378295,26.));
#127331=CARTESIAN_POINT('Origin',(13.7005576038968,42.6304565378295,26.));
#127332=CARTESIAN_POINT('',(13.7005576038968,43.1304565378295,26.));
#127333=CARTESIAN_POINT('',(13.7005576038968,43.1304565378295,26.));
#127334=CARTESIAN_POINT('Origin',(13.7005576038968,42.6304565378295,26.));
#127335=CARTESIAN_POINT('Origin',(12.8005576038968,43.1304565378295,26.));
#127336=CARTESIAN_POINT('',(12.8005576038968,43.1304565378295,26.));
#127337=CARTESIAN_POINT('Origin',(12.5005576038968,44.8304565378295,26.));
#127338=CARTESIAN_POINT('',(12.5005576038968,44.8304565378295,26.));
#127339=CARTESIAN_POINT('',(12.5005576038968,44.8304565378295,26.));
#127340=CARTESIAN_POINT('',(12.5005576038968,44.8304565378295,106.));
#127341=CARTESIAN_POINT('',(12.5005576038968,44.8304565378295,106.));
#127342=CARTESIAN_POINT('',(12.5005576038968,44.8304565378295,26.));
#127343=CARTESIAN_POINT('Origin',(12.8005576038968,44.8304565378295,26.));
#127344=CARTESIAN_POINT('',(12.8005576038968,45.1304565378295,26.));
#127345=CARTESIAN_POINT('Origin',(12.8005576038968,44.8304565378295,26.));
#127346=CARTESIAN_POINT('',(12.8005576038968,45.1304565378295,106.));
#127347=CARTESIAN_POINT('Origin',(12.8005576038968,44.8304565378295,106.));
#127348=CARTESIAN_POINT('',(12.8005576038968,45.1304565378295,26.));
#127349=CARTESIAN_POINT('Origin',(15.5005576038968,45.1304565378295,26.));
#127350=CARTESIAN_POINT('',(15.5005576038968,45.1304565378295,26.));
#127351=CARTESIAN_POINT('',(15.5005576038968,45.1304565378295,26.));
#127352=CARTESIAN_POINT('',(15.5005576038968,45.1304565378295,106.));
#127353=CARTESIAN_POINT('',(15.5005576038968,45.1304565378295,106.));
#127354=CARTESIAN_POINT('',(15.5005576038968,45.1304565378295,26.));
#127355=CARTESIAN_POINT('Origin',(15.5005576038968,44.6304565378295,26.));
#127356=CARTESIAN_POINT('',(16.0005576038968,44.6304565378295,26.));
#127357=CARTESIAN_POINT('Origin',(15.5005576038968,44.6304565378295,26.));
#127358=CARTESIAN_POINT('',(16.0005576038968,44.6304565378295,106.));
#127359=CARTESIAN_POINT('Origin',(15.5005576038968,44.6304565378295,106.));
#127360=CARTESIAN_POINT('',(16.0005576038968,44.6304565378295,26.));
#127361=CARTESIAN_POINT('Origin',(16.0005576038968,36.1384565378295,26.));
#127362=CARTESIAN_POINT('',(16.0005576038968,36.1384565378295,26.));
#127363=CARTESIAN_POINT('',(16.0005576038968,36.1384565378295,26.));
#127364=CARTESIAN_POINT('',(16.0005576038968,36.1384565378295,106.));
#127365=CARTESIAN_POINT('',(16.0005576038968,36.1384565378295,106.));
#127366=CARTESIAN_POINT('',(16.0005576038968,36.1384565378295,26.));
#127367=CARTESIAN_POINT('Origin',(16.5085576038968,36.1384565378295,26.));
#127368=CARTESIAN_POINT('',(16.5085576038968,35.6304565378295,26.));
#127369=CARTESIAN_POINT('Origin',(16.5085576038968,36.1384565378295,26.));
#127370=CARTESIAN_POINT('',(16.5085576038968,35.6304565378295,106.));
#127371=CARTESIAN_POINT('Origin',(16.5085576038968,36.1384565378295,106.));
#127372=CARTESIAN_POINT('',(16.5085576038968,35.6304565378295,26.));
#127373=CARTESIAN_POINT('Origin',(16.8285576038968,35.6304565378295,26.));
#127374=CARTESIAN_POINT('',(16.8285576038968,35.6304565378295,26.));
#127375=CARTESIAN_POINT('',(16.8285576038968,35.6304565378295,26.));
#127376=CARTESIAN_POINT('',(16.8285576038968,35.6304565378295,106.));
#127377=CARTESIAN_POINT('',(16.8285576038968,35.6304565378295,106.));
#127378=CARTESIAN_POINT('',(16.8285576038968,35.6304565378295,26.));
#127379=CARTESIAN_POINT('Origin',(16.8285576038968,32.6304565378295,26.));
#127380=CARTESIAN_POINT('',(18.9498779474565,34.7517768813891,26.));
#127381=CARTESIAN_POINT('Origin',(16.8285576038968,32.6304565378295,26.));
#127382=CARTESIAN_POINT('',(18.9498779474565,34.7517768813891,106.));
#127383=CARTESIAN_POINT('Origin',(16.8285576038968,32.6304565378295,106.));
#127384=CARTESIAN_POINT('',(18.9498779474565,34.7517768813891,26.));
#127385=CARTESIAN_POINT('Origin',(24.535314412049,29.1663404167966,26.));
#127386=CARTESIAN_POINT('',(24.535314412049,29.1663404167966,26.));
#127387=CARTESIAN_POINT('',(24.535314412049,29.1663404167966,26.));
#127388=CARTESIAN_POINT('',(24.535314412049,29.1663404167966,106.));
#127389=CARTESIAN_POINT('',(24.535314412049,29.1663404167966,106.));
#127390=CARTESIAN_POINT('',(24.535314412049,29.1663404167966,26.));
#127391=CARTESIAN_POINT('Origin',(20.9997805061163,25.6308065108639,26.));
#127392=CARTESIAN_POINT('',(25.9997805061163,25.6308065108639,26.));
#127393=CARTESIAN_POINT('Origin',(20.9997805061163,25.6308065108639,26.));
#127394=CARTESIAN_POINT('',(25.9997805061163,25.6308065108639,106.));
#127395=CARTESIAN_POINT('Origin',(20.9997805061163,25.6308065108639,106.));
#127396=CARTESIAN_POINT('',(25.9997805061163,25.6308065108639,26.));
#127397=CARTESIAN_POINT('Origin',(25.9997805061163,12.1308065108639,26.));
#127398=CARTESIAN_POINT('',(25.9997805061163,12.1308065108639,26.));
#127399=CARTESIAN_POINT('',(25.9997805061163,12.1308065108639,26.));
#127400=CARTESIAN_POINT('',(25.9997805061163,12.1308065108639,106.));
#127401=CARTESIAN_POINT('',(25.9997805061163,12.1308065108639,106.));
#127402=CARTESIAN_POINT('',(25.9997805061163,12.1308065108639,26.));
#127403=CARTESIAN_POINT('Origin',(24.9997805061163,12.1308065108639,26.));
#127404=CARTESIAN_POINT('',(24.9997805061163,11.1308065108639,26.));
#127405=CARTESIAN_POINT('Origin',(24.9997805061163,12.1308065108639,26.));
#127406=CARTESIAN_POINT('',(24.9997805061163,11.1308065108639,106.));
#127407=CARTESIAN_POINT('Origin',(24.9997805061163,12.1308065108639,106.));
#127408=CARTESIAN_POINT('',(24.9997805061163,11.1308065108639,26.));
#127409=CARTESIAN_POINT('Origin',(20.4997805061163,11.1308065108639,26.));
#127410=CARTESIAN_POINT('',(20.4997805061163,11.1308065108639,26.));
#127411=CARTESIAN_POINT('',(20.4997805061163,11.1308065108639,26.));
#127412=CARTESIAN_POINT('',(20.4997805061163,11.1308065108639,106.));
#127413=CARTESIAN_POINT('',(20.4997805061163,11.1308065108639,106.));
#127414=CARTESIAN_POINT('',(20.4997805061163,11.1308065108639,26.));
#127415=CARTESIAN_POINT('Origin',(19.0000070232196,12.6305799937605,26.));
#127416=CARTESIAN_POINT('',(19.0000070232196,12.6305799937605,26.));
#127417=CARTESIAN_POINT('',(19.0000070232196,12.6305799937605,26.));
#127418=CARTESIAN_POINT('',(19.0000070232196,12.6305799937605,106.));
#127419=CARTESIAN_POINT('',(19.0000070232196,12.6305799937605,106.));
#127420=CARTESIAN_POINT('',(19.0000070232196,12.6305799937605,26.));
#127421=CARTESIAN_POINT('Origin',(19.0000070232196,21.8015799937605,26.));
#127422=CARTESIAN_POINT('',(19.0000070232196,21.8015799937605,26.));
#127423=CARTESIAN_POINT('',(19.0000070232196,21.8015799937605,26.));
#127424=CARTESIAN_POINT('',(19.0000070232196,21.8015799937605,106.));
#127425=CARTESIAN_POINT('',(19.0000070232196,21.8015799937605,106.));
#127426=CARTESIAN_POINT('',(19.0000070232196,21.8015799937605,26.));
#127427=CARTESIAN_POINT('Origin',(18.0000070232196,21.8015799937605,26.));
#127428=CARTESIAN_POINT('',(18.4694785860055,22.6845275866195,26.));
#127429=CARTESIAN_POINT('Origin',(18.0000070232196,21.8015799937605,26.));
#127430=CARTESIAN_POINT('',(18.4694785860055,22.6845275866195,106.));
#127431=CARTESIAN_POINT('Origin',(18.0000070232196,21.8015799937605,106.));
#127432=CARTESIAN_POINT('',(18.4694785860055,22.6845275866195,26.));
#127433=CARTESIAN_POINT('Origin',(15.75,24.1305,26.));
#127434=CARTESIAN_POINT('',(15.75,24.1305,26.));
#127435=CARTESIAN_POINT('',(15.75,24.1305,26.));
#127436=CARTESIAN_POINT('',(15.75,24.1305,106.));
#127437=CARTESIAN_POINT('',(15.75,24.1305,106.));
#127438=CARTESIAN_POINT('',(15.75,24.1305,26.));
#127439=CARTESIAN_POINT('Origin',(12.,24.1305,26.));
#127440=CARTESIAN_POINT('',(12.,24.1305,26.));
#127441=CARTESIAN_POINT('',(12.,24.1305,26.));
#127442=CARTESIAN_POINT('',(12.,24.1305,106.));
#127443=CARTESIAN_POINT('',(12.,24.1305,106.));
#127444=CARTESIAN_POINT('',(12.,24.1305,26.));
#127445=CARTESIAN_POINT('Origin',(12.,30.5305,26.));
#127446=CARTESIAN_POINT('',(12.,30.5305,26.));
#127447=CARTESIAN_POINT('',(12.,30.5305,106.));
#127448=CARTESIAN_POINT('Origin',(12.9998902530581,28.1306315243467,106.));
#127449=CARTESIAN_POINT('Origin',(12.9998902530581,28.1306315243467,26.));
#127450=CARTESIAN_POINT('',(0.,0.,0.));
#127451=CARTESIAN_POINT('',(0.,0.,132.));
#215592=UNCERTAINTY_MEASURE_WITH_UNIT(LENGTH_MEASURE(0.01),#215610,
'DISTANCE_ACCURACY_VALUE',
'Maximum model space distance between geometric entities at asserted c
onnectivities');
#215598=UNCERTAINTY_MEASURE_WITH_UNIT(LENGTH_MEASURE(0.01),#215610,
'DISTANCE_ACCURACY_VALUE',
'Maximum model space distance between geometric entities at asserted c
onnectivities');
#215603=(
GEOMETRIC_REPRESENTATION_CONTEXT(3)
GLOBAL_UNCERTAINTY_ASSIGNED_CONTEXT((#215592))
GLOBAL_UNIT_ASSIGNED_CONTEXT((#215610,#215612,#215613))
REPRESENTATION_CONTEXT('','3D')
);
#215609=(
GEOMETRIC_REPRESENTATION_CONTEXT(3)
GLOBAL_UNCERTAINTY_ASSIGNED_CONTEXT((#215598))
GLOBAL_UNIT_ASSIGNED_CONTEXT((#215610,#215612,#215613))
REPRESENTATION_CONTEXT('','3D')
);
#215610=(
LENGTH_UNIT()
NAMED_UNIT(*)
SI_UNIT(.MILLI.,.METRE.)
);
#215612=(
NAMED_UNIT(*)
PLANE_ANGLE_UNIT()
SI_UNIT($,.RADIAN.)
);
#215613=(
NAMED_UNIT(*)
SI_UNIT($,.STERADIAN.)
SOLID_ANGLE_UNIT()
);
#215618=SHAPE_DEFINITION_REPRESENTATION(#215628,#215647);
#215628=PRODUCT_DEFINITION_SHAPE('',$,#215658);
#215647=SHAPE_REPRESENTATION('',(#28709,#29431,#29432),#215603);
#215653=PRODUCT_DEFINITION_CONTEXT('part definition',#215685,'design');
#215658=PRODUCT_DEFINITION('2026-10-04-15-17-49-077','Carriage',#215668,
#215653);
#215668=PRODUCT_DEFINITION_FORMATION('',$,#215691);
#215685=APPLICATION_CONTEXT(
'Core Data for Automotive Mechanical Design Process');
#215686=PRODUCT_CONTEXT('part definition',#215685,'mechanical');
#215691=PRODUCT('2026-10-04-15-17-49-077','Carriage',$,(#215686));
#215698=PRESENTATION_STYLE_ASSIGNMENT((#215700));
#215700=SURFACE_STYLE_USAGE(.BOTH.,#215702);
#215702=SURFACE_SIDE_STYLE('',(#215704));
#215704=SURFACE_STYLE_FILL_AREA(#215706);
#215706=FILL_AREA_STYLE('Opaque(245,245,246)',(#215708));
#215708=FILL_AREA_STYLE_COLOUR('Opaque(245,245,246)',#215710);
#215710=COLOUR_RGB('Opaque(245,245,246)', 0.66274510, 0.83137255, 0.94901961);
ENDSEC;
END-ISO-10303-21;
